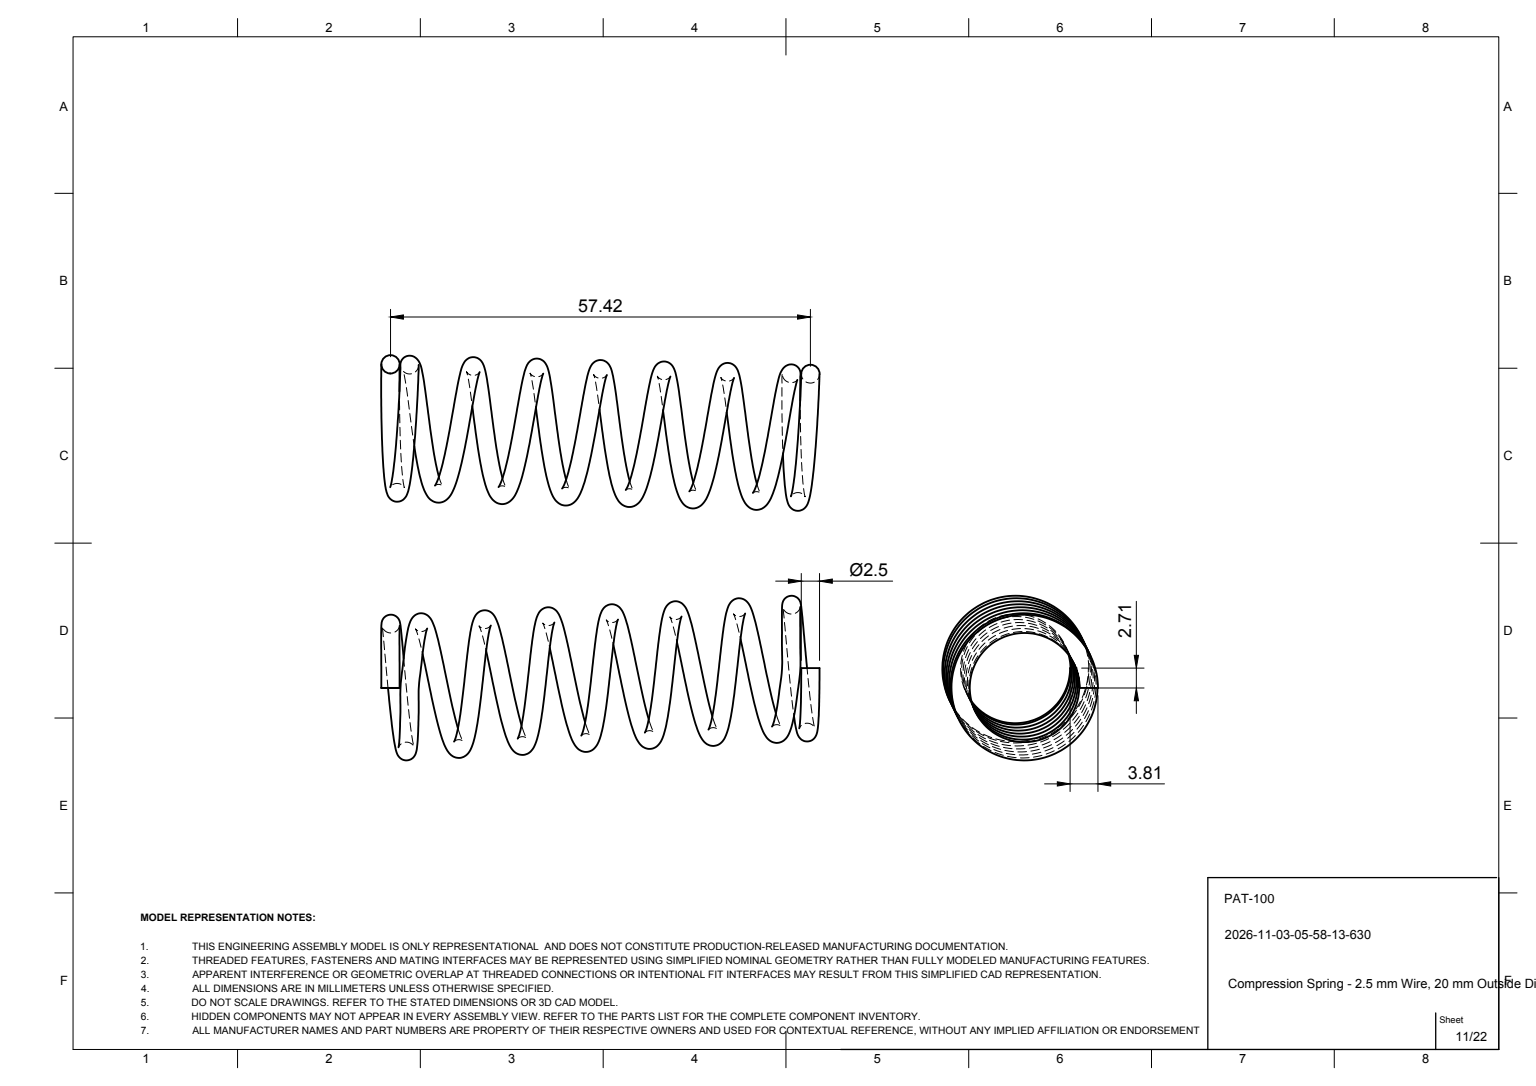
ISO-10303-21;
HEADER;
/* Generated by software containing ST-Developer
 * from STEP Tools, Inc. (www.steptools.com) 
 */

FILE_DESCRIPTION(
/* description */ (''),
/* implementation_level */ '2;1');

FILE_NAME(
/* name */ 'Compression Spring - 2.5 mm Wire, 20 mm Outside Diameter, 60 mm Long.step',
/* time_stamp */ '2026-10-29T16:43:51-07:00',
/* author */ (''),
/* organization */ (''),
/* preprocessor_version */ 'ST-DEVELOPER v20.2',
/* originating_system */ 'Autodesk Translation Framework v15.17.0.0',
/* authorisation */ '');

FILE_SCHEMA (('AUTOMOTIVE_DESIGN { 1 0 10303 214 3 1 1 }'));
ENDSEC;

DATA;
#10=MECHANICAL_DESIGN_GEOMETRIC_PRESENTATION_REPRESENTATION('',(#375),#10292);
#259=B_SPLINE_CURVE_WITH_KNOTS('',3,(#9348,#9349,#9350,#9351,#9352,#9353,
#9354,#9355,#9356,#9357,#9358,#9359,#9360,#9361,#9362,#9363,#9364,#9365,
#9366,#9367,#9368,#9369,#9370,#9371,#9372,#9373,#9374,#9375,#9376,#9377,
#9378,#9379,#9380,#9381,#9382,#9383,#9384,#9385,#9386,#9387,#9388,#9389,
#9390,#9391,#9392,#9393,#9394,#9395,#9396,#9397,#9398,#9399,#9400,#9401,
#9402,#9403,#9404,#9405,#9406,#9407,#9408,#9409,#9410,#9411,#9412,#9413,
#9414,#9415,#9416,#9417,#9418,#9419,#9420,#9421,#9422,#9423,#9424,#9425,
#9426,#9427,#9428,#9429,#9430,#9431,#9432,#9433,#9434,#9435,#9436,#9437,
#9438,#9439,#9440,#9441,#9442,#9443,#9444,#9445,#9446,#9447,#9448,#9449,
#9450,#9451,#9452,#9453,#9454,#9455,#9456,#9457,#9458,#9459,#9460,#9461,
#9462,#9463,#9464,#9465,#9466,#9467,#9468,#9469,#9470),.UNSPECIFIED.,.F.,
 .F.,(4,1,1,1,1,1,1,1,1,1,1,1,1,1,1,1,1,1,1,1,1,1,1,1,1,1,1,1,1,1,1,1,1,
1,1,1,1,1,1,1,1,1,1,1,1,1,1,1,1,1,1,1,1,1,1,1,1,1,1,1,1,1,1,1,1,1,1,1,1,
1,1,1,1,1,1,1,1,1,1,1,1,1,1,1,1,1,1,1,1,1,1,1,1,1,1,1,1,1,1,1,1,1,1,1,1,
1,1,1,1,1,1,1,1,1,1,1,1,1,1,1,4),(0.,0.00446428571428571,0.00892857142857143,
0.0178571428571429,0.0267857142857143,0.0357142857142857,0.0446428571428571,
0.0535714285714286,0.0625,0.0714285714285714,0.0803571428571428,0.0892857142857143,
0.0982142857142857,0.107142857142857,0.111607142857143,0.116071428571429,
0.120535714285714,0.122767857142857,0.125,0.129464285714286,0.133928571428571,
0.138392857142857,0.142857142857143,0.151785714285714,0.160714285714286,
0.169642857142857,0.174107142857143,0.178571428571429,0.1875,0.196428571428571,
0.205357142857143,0.214285714285714,0.223214285714286,0.232142857142857,
0.241071428571429,0.25,0.258928571428571,0.267857142857143,0.276785714285714,
0.285714285714286,0.294642857142857,0.303571428571429,0.3125,0.321428571428571,
0.330357142857143,0.339285714285714,0.348214285714286,0.357142857142857,
0.363095238095238,0.369047619047619,0.380952380952381,0.392857142857143,
0.401785714285714,0.410714285714286,0.419642857142857,0.428571428571429,
0.4375,0.446428571428571,0.455357142857143,0.464285714285714,0.476190476190476,
0.488095238095238,0.5,0.508928571428571,0.517857142857143,0.526785714285714,
0.535714285714286,0.544642857142857,0.553571428571429,0.5625,0.571428571428571,
0.580357142857143,0.589285714285714,0.598214285714286,0.607142857142857,
0.616071428571429,0.625,0.633928571428571,0.642857142857143,0.654761904761905,
0.666666666666667,0.678571428571428,0.6875,0.696428571428571,0.705357142857143,
0.714285714285714,0.720238095238095,0.726190476190476,0.738095238095238,
0.75,0.761904761904762,0.773809523809524,0.785714285714286,0.797619047619047,
0.809523809523809,0.821428571428571,0.833333333333333,0.845238095238095,
0.857142857142857,0.861607142857143,0.866071428571429,0.870535714285714,
0.875,0.877232142857143,0.879464285714286,0.883928571428571,0.888392857142857,
0.892857142857143,0.901785714285714,0.910714285714286,0.919642857142857,
0.928571428571429,0.9375,0.946428571428571,0.955357142857143,0.964285714285714,
0.973214285714286,0.982142857142857,0.991071428571429,0.995535714285714,
1.),.UNSPECIFIED.);
#264=B_SPLINE_SURFACE_WITH_KNOTS('',3,3,((#8115,#8116,#8117,#8118,#8119,
#8120,#8121,#8122,#8123,#8124,#8125,#8126,#8127,#8128,#8129,#8130,#8131,
#8132,#8133,#8134,#8135,#8136,#8137,#8138,#8139,#8140,#8141,#8142,#8143,
#8144,#8145,#8146,#8147,#8148,#8149,#8150,#8151,#8152,#8153,#8154,#8155,
#8156,#8157,#8158,#8159,#8160,#8161,#8162,#8163,#8164,#8165,#8166,#8167,
#8168,#8169,#8170,#8171,#8172,#8173,#8174,#8175,#8176,#8177,#8178,#8179,
#8180,#8181,#8182,#8183,#8184,#8185,#8186,#8187,#8188,#8189,#8190,#8191,
#8192,#8193,#8194,#8195,#8196,#8197,#8198,#8199,#8200,#8201,#8202,#8203,
#8204,#8205,#8206,#8207,#8208,#8209,#8210,#8211,#8212,#8213,#8214,#8215,
#8216,#8217,#8218,#8219,#8220,#8221,#8222,#8223,#8224,#8225,#8226,#8227,
#8228,#8229,#8230,#8231,#8232,#8233,#8234,#8235,#8236,#8237),(#8238,#8239,
#8240,#8241,#8242,#8243,#8244,#8245,#8246,#8247,#8248,#8249,#8250,#8251,
#8252,#8253,#8254,#8255,#8256,#8257,#8258,#8259,#8260,#8261,#8262,#8263,
#8264,#8265,#8266,#8267,#8268,#8269,#8270,#8271,#8272,#8273,#8274,#8275,
#8276,#8277,#8278,#8279,#8280,#8281,#8282,#8283,#8284,#8285,#8286,#8287,
#8288,#8289,#8290,#8291,#8292,#8293,#8294,#8295,#8296,#8297,#8298,#8299,
#8300,#8301,#8302,#8303,#8304,#8305,#8306,#8307,#8308,#8309,#8310,#8311,
#8312,#8313,#8314,#8315,#8316,#8317,#8318,#8319,#8320,#8321,#8322,#8323,
#8324,#8325,#8326,#8327,#8328,#8329,#8330,#8331,#8332,#8333,#8334,#8335,
#8336,#8337,#8338,#8339,#8340,#8341,#8342,#8343,#8344,#8345,#8346,#8347,
#8348,#8349,#8350,#8351,#8352,#8353,#8354,#8355,#8356,#8357,#8358,#8359,
#8360),(#8361,#8362,#8363,#8364,#8365,#8366,#8367,#8368,#8369,#8370,#8371,
#8372,#8373,#8374,#8375,#8376,#8377,#8378,#8379,#8380,#8381,#8382,#8383,
#8384,#8385,#8386,#8387,#8388,#8389,#8390,#8391,#8392,#8393,#8394,#8395,
#8396,#8397,#8398,#8399,#8400,#8401,#8402,#8403,#8404,#8405,#8406,#8407,
#8408,#8409,#8410,#8411,#8412,#8413,#8414,#8415,#8416,#8417,#8418,#8419,
#8420,#8421,#8422,#8423,#8424,#8425,#8426,#8427,#8428,#8429,#8430,#8431,
#8432,#8433,#8434,#8435,#8436,#8437,#8438,#8439,#8440,#8441,#8442,#8443,
#8444,#8445,#8446,#8447,#8448,#8449,#8450,#8451,#8452,#8453,#8454,#8455,
#8456,#8457,#8458,#8459,#8460,#8461,#8462,#8463,#8464,#8465,#8466,#8467,
#8468,#8469,#8470,#8471,#8472,#8473,#8474,#8475,#8476,#8477,#8478,#8479,
#8480,#8481,#8482,#8483),(#8484,#8485,#8486,#8487,#8488,#8489,#8490,#8491,
#8492,#8493,#8494,#8495,#8496,#8497,#8498,#8499,#8500,#8501,#8502,#8503,
#8504,#8505,#8506,#8507,#8508,#8509,#8510,#8511,#8512,#8513,#8514,#8515,
#8516,#8517,#8518,#8519,#8520,#8521,#8522,#8523,#8524,#8525,#8526,#8527,
#8528,#8529,#8530,#8531,#8532,#8533,#8534,#8535,#8536,#8537,#8538,#8539,
#8540,#8541,#8542,#8543,#8544,#8545,#8546,#8547,#8548,#8549,#8550,#8551,
#8552,#8553,#8554,#8555,#8556,#8557,#8558,#8559,#8560,#8561,#8562,#8563,
#8564,#8565,#8566,#8567,#8568,#8569,#8570,#8571,#8572,#8573,#8574,#8575,
#8576,#8577,#8578,#8579,#8580,#8581,#8582,#8583,#8584,#8585,#8586,#8587,
#8588,#8589,#8590,#8591,#8592,#8593,#8594,#8595,#8596,#8597,#8598,#8599,
#8600,#8601,#8602,#8603,#8604,#8605,#8606),(#8607,#8608,#8609,#8610,#8611,
#8612,#8613,#8614,#8615,#8616,#8617,#8618,#8619,#8620,#8621,#8622,#8623,
#8624,#8625,#8626,#8627,#8628,#8629,#8630,#8631,#8632,#8633,#8634,#8635,
#8636,#8637,#8638,#8639,#8640,#8641,#8642,#8643,#8644,#8645,#8646,#8647,
#8648,#8649,#8650,#8651,#8652,#8653,#8654,#8655,#8656,#8657,#8658,#8659,
#8660,#8661,#8662,#8663,#8664,#8665,#8666,#8667,#8668,#8669,#8670,#8671,
#8672,#8673,#8674,#8675,#8676,#8677,#8678,#8679,#8680,#8681,#8682,#8683,
#8684,#8685,#8686,#8687,#8688,#8689,#8690,#8691,#8692,#8693,#8694,#8695,
#8696,#8697,#8698,#8699,#8700,#8701,#8702,#8703,#8704,#8705,#8706,#8707,
#8708,#8709,#8710,#8711,#8712,#8713,#8714,#8715,#8716,#8717,#8718,#8719,
#8720,#8721,#8722,#8723,#8724,#8725,#8726,#8727,#8728,#8729),(#8730,#8731,
#8732,#8733,#8734,#8735,#8736,#8737,#8738,#8739,#8740,#8741,#8742,#8743,
#8744,#8745,#8746,#8747,#8748,#8749,#8750,#8751,#8752,#8753,#8754,#8755,
#8756,#8757,#8758,#8759,#8760,#8761,#8762,#8763,#8764,#8765,#8766,#8767,
#8768,#8769,#8770,#8771,#8772,#8773,#8774,#8775,#8776,#8777,#8778,#8779,
#8780,#8781,#8782,#8783,#8784,#8785,#8786,#8787,#8788,#8789,#8790,#8791,
#8792,#8793,#8794,#8795,#8796,#8797,#8798,#8799,#8800,#8801,#8802,#8803,
#8804,#8805,#8806,#8807,#8808,#8809,#8810,#8811,#8812,#8813,#8814,#8815,
#8816,#8817,#8818,#8819,#8820,#8821,#8822,#8823,#8824,#8825,#8826,#8827,
#8828,#8829,#8830,#8831,#8832,#8833,#8834,#8835,#8836,#8837,#8838,#8839,
#8840,#8841,#8842,#8843,#8844,#8845,#8846,#8847,#8848,#8849,#8850,#8851,
#8852),(#8853,#8854,#8855,#8856,#8857,#8858,#8859,#8860,#8861,#8862,#8863,
#8864,#8865,#8866,#8867,#8868,#8869,#8870,#8871,#8872,#8873,#8874,#8875,
#8876,#8877,#8878,#8879,#8880,#8881,#8882,#8883,#8884,#8885,#8886,#8887,
#8888,#8889,#8890,#8891,#8892,#8893,#8894,#8895,#8896,#8897,#8898,#8899,
#8900,#8901,#8902,#8903,#8904,#8905,#8906,#8907,#8908,#8909,#8910,#8911,
#8912,#8913,#8914,#8915,#8916,#8917,#8918,#8919,#8920,#8921,#8922,#8923,
#8924,#8925,#8926,#8927,#8928,#8929,#8930,#8931,#8932,#8933,#8934,#8935,
#8936,#8937,#8938,#8939,#8940,#8941,#8942,#8943,#8944,#8945,#8946,#8947,
#8948,#8949,#8950,#8951,#8952,#8953,#8954,#8955,#8956,#8957,#8958,#8959,
#8960,#8961,#8962,#8963,#8964,#8965,#8966,#8967,#8968,#8969,#8970,#8971,
#8972,#8973,#8974,#8975),(#8976,#8977,#8978,#8979,#8980,#8981,#8982,#8983,
#8984,#8985,#8986,#8987,#8988,#8989,#8990,#8991,#8992,#8993,#8994,#8995,
#8996,#8997,#8998,#8999,#9000,#9001,#9002,#9003,#9004,#9005,#9006,#9007,
#9008,#9009,#9010,#9011,#9012,#9013,#9014,#9015,#9016,#9017,#9018,#9019,
#9020,#9021,#9022,#9023,#9024,#9025,#9026,#9027,#9028,#9029,#9030,#9031,
#9032,#9033,#9034,#9035,#9036,#9037,#9038,#9039,#9040,#9041,#9042,#9043,
#9044,#9045,#9046,#9047,#9048,#9049,#9050,#9051,#9052,#9053,#9054,#9055,
#9056,#9057,#9058,#9059,#9060,#9061,#9062,#9063,#9064,#9065,#9066,#9067,
#9068,#9069,#9070,#9071,#9072,#9073,#9074,#9075,#9076,#9077,#9078,#9079,
#9080,#9081,#9082,#9083,#9084,#9085,#9086,#9087,#9088,#9089,#9090,#9091,
#9092,#9093,#9094,#9095,#9096,#9097,#9098),(#9099,#9100,#9101,#9102,#9103,
#9104,#9105,#9106,#9107,#9108,#9109,#9110,#9111,#9112,#9113,#9114,#9115,
#9116,#9117,#9118,#9119,#9120,#9121,#9122,#9123,#9124,#9125,#9126,#9127,
#9128,#9129,#9130,#9131,#9132,#9133,#9134,#9135,#9136,#9137,#9138,#9139,
#9140,#9141,#9142,#9143,#9144,#9145,#9146,#9147,#9148,#9149,#9150,#9151,
#9152,#9153,#9154,#9155,#9156,#9157,#9158,#9159,#9160,#9161,#9162,#9163,
#9164,#9165,#9166,#9167,#9168,#9169,#9170,#9171,#9172,#9173,#9174,#9175,
#9176,#9177,#9178,#9179,#9180,#9181,#9182,#9183,#9184,#9185,#9186,#9187,
#9188,#9189,#9190,#9191,#9192,#9193,#9194,#9195,#9196,#9197,#9198,#9199,
#9200,#9201,#9202,#9203,#9204,#9205,#9206,#9207,#9208,#9209,#9210,#9211,
#9212,#9213,#9214,#9215,#9216,#9217,#9218,#9219,#9220,#9221),(#9222,#9223,
#9224,#9225,#9226,#9227,#9228,#9229,#9230,#9231,#9232,#9233,#9234,#9235,
#9236,#9237,#9238,#9239,#9240,#9241,#9242,#9243,#9244,#9245,#9246,#9247,
#9248,#9249,#9250,#9251,#9252,#9253,#9254,#9255,#9256,#9257,#9258,#9259,
#9260,#9261,#9262,#9263,#9264,#9265,#9266,#9267,#9268,#9269,#9270,#9271,
#9272,#9273,#9274,#9275,#9276,#9277,#9278,#9279,#9280,#9281,#9282,#9283,
#9284,#9285,#9286,#9287,#9288,#9289,#9290,#9291,#9292,#9293,#9294,#9295,
#9296,#9297,#9298,#9299,#9300,#9301,#9302,#9303,#9304,#9305,#9306,#9307,
#9308,#9309,#9310,#9311,#9312,#9313,#9314,#9315,#9316,#9317,#9318,#9319,
#9320,#9321,#9322,#9323,#9324,#9325,#9326,#9327,#9328,#9329,#9330,#9331,
#9332,#9333,#9334,#9335,#9336,#9337,#9338,#9339,#9340,#9341,#9342,#9343,
#9344)),.UNSPECIFIED.,.T.,.F.,.F.,(4,1,1,1,1,1,1,4),(4,1,1,1,1,1,1,1,1,
1,1,1,1,1,1,1,1,1,1,1,1,1,1,1,1,1,1,1,1,1,1,1,1,1,1,1,1,1,1,1,1,1,1,1,1,
1,1,1,1,1,1,1,1,1,1,1,1,1,1,1,1,1,1,1,1,1,1,1,1,1,1,1,1,1,1,1,1,1,1,1,1,
1,1,1,1,1,1,1,1,1,1,1,1,1,1,1,1,1,1,1,1,1,1,1,1,1,1,1,1,1,1,1,1,1,1,1,1,
1,1,1,4),(-3.14159265358979,-2.24399475256414,-1.34639685153848,-0.448798950512828,
0.448798950512828,1.34639685153848,2.24399475256414,3.14159265358979),(0.,
0.00446428571428571,0.00892857142857143,0.0178571428571429,0.0267857142857143,
0.0357142857142857,0.0446428571428571,0.0535714285714286,0.0625,0.0714285714285714,
0.0803571428571428,0.0892857142857143,0.0982142857142857,0.107142857142857,
0.111607142857143,0.116071428571429,0.120535714285714,0.122767857142857,
0.125,0.129464285714286,0.133928571428571,0.138392857142857,0.142857142857143,
0.151785714285714,0.160714285714286,0.169642857142857,0.174107142857143,
0.178571428571429,0.1875,0.196428571428571,0.205357142857143,0.214285714285714,
0.223214285714286,0.232142857142857,0.241071428571429,0.25,0.258928571428571,
0.267857142857143,0.276785714285714,0.285714285714286,0.294642857142857,
0.303571428571429,0.3125,0.321428571428571,0.330357142857143,0.339285714285714,
0.348214285714286,0.357142857142857,0.363095238095238,0.369047619047619,
0.380952380952381,0.392857142857143,0.401785714285714,0.410714285714286,
0.419642857142857,0.428571428571429,0.4375,0.446428571428571,0.455357142857143,
0.464285714285714,0.476190476190476,0.488095238095238,0.5,0.508928571428571,
0.517857142857143,0.526785714285714,0.535714285714286,0.544642857142857,
0.553571428571429,0.5625,0.571428571428571,0.580357142857143,0.589285714285714,
0.598214285714286,0.607142857142857,0.616071428571429,0.625,0.633928571428571,
0.642857142857143,0.654761904761905,0.666666666666667,0.678571428571428,
0.6875,0.696428571428571,0.705357142857143,0.714285714285714,0.720238095238095,
0.726190476190476,0.738095238095238,0.75,0.761904761904762,0.773809523809524,
0.785714285714286,0.797619047619047,0.809523809523809,0.821428571428571,
0.833333333333333,0.845238095238095,0.857142857142857,0.861607142857143,
0.866071428571429,0.870535714285714,0.875,0.877232142857143,0.879464285714286,
0.883928571428571,0.888392857142857,0.892857142857143,0.901785714285714,
0.910714285714286,0.919642857142857,0.928571428571429,0.9375,0.946428571428571,
0.955357142857143,0.964285714285714,0.973214285714286,0.982142857142857,
0.991071428571429,0.995535714285714,1.),.UNSPECIFIED.);
#329=SHAPE_REPRESENTATION_RELATIONSHIP('SRR','None',#10425,#352);
#352=ADVANCED_BREP_SHAPE_REPRESENTATION('',(#396),#10277);
#375=STYLED_ITEM('',(#10628),#396);
#396=MANIFOLD_SOLID_BREP('Body1',#5019);
#619=PLANE('',#5533);
#620=PLANE('',#5534);
#849=FACE_OUTER_BOUND('',#1201,.T.);
#850=FACE_OUTER_BOUND('',#1202,.T.);
#851=FACE_OUTER_BOUND('',#1203,.T.);
#1201=EDGE_LOOP('',(#4039,#4040,#4041,#4042));
#1202=EDGE_LOOP('',(#4043));
#1203=EDGE_LOOP('',(#4044));
#2285=CIRCLE('',#5531,0.125);
#2286=CIRCLE('',#5532,0.125);
#2600=VERTEX_POINT('',#9345);
#2601=VERTEX_POINT('',#9347);
#3110=EDGE_CURVE('',#2600,#2600,#2285,.T.);
#3111=EDGE_CURVE('',#2600,#2601,#259,.T.);
#3112=EDGE_CURVE('',#2601,#2601,#2286,.T.);
#4039=ORIENTED_EDGE('',*,*,#3110,.T.);
#4040=ORIENTED_EDGE('',*,*,#3111,.T.);
#4041=ORIENTED_EDGE('',*,*,#3112,.F.);
#4042=ORIENTED_EDGE('',*,*,#3111,.F.);
#4043=ORIENTED_EDGE('',*,*,#3112,.T.);
#4044=ORIENTED_EDGE('',*,*,#3110,.F.);
#4858=ADVANCED_FACE('',(#849),#264,.T.);
#4859=ADVANCED_FACE('',(#850),#619,.T.);
#4860=ADVANCED_FACE('',(#851),#620,.F.);
#5019=CLOSED_SHELL('',(#4858,#4859,#4860));
#5530=AXIS2_PLACEMENT_3D('',#8114,#6553,#6554);
#5531=AXIS2_PLACEMENT_3D('',#9346,#6555,#6556);
#5532=AXIS2_PLACEMENT_3D('',#9471,#6557,#6558);
#5533=AXIS2_PLACEMENT_3D('',#9472,#6559,#6560);
#5534=AXIS2_PLACEMENT_3D('',#9473,#6561,#6562);
#6553=DIRECTION('axis',(0.,0.,1.));
#6554=DIRECTION('refdir',(1.,0.,0.));
#6555=DIRECTION('center_axis',(-0.00107151163471255,0.0471293712697611,
0.998888219084865));
#6556=DIRECTION('ref_axis',(0.022704394310356,-0.998630154113891,0.0471415503931119));
#6557=DIRECTION('center_axis',(0.0010715115821705,0.0471293712204561,0.998888219087248));
#6558=DIRECTION('ref_axis',(0.234516922063796,-0.971043629832377,0.045564045339339));
#6559=DIRECTION('center_axis',(0.0010715115821705,0.0471293712204561,0.998888219087248));
#6560=DIRECTION('ref_axis',(0.234516922063796,-0.971043629832377,0.045564045339339));
#6561=DIRECTION('center_axis',(-0.00107151163471255,0.0471293712697611,
0.998888219084865));
#6562=DIRECTION('ref_axis',(0.022704394310356,-0.998630154113891,0.0471415503931119));
#8114=CARTESIAN_POINT('',(0.,0.,0.));
#8115=CARTESIAN_POINT('Ctrl Pts',(0.872161950711206,0.124828769264236,-0.00589269379913899));
#8116=CARTESIAN_POINT('Ctrl Pts',(0.872090904698941,0.127953657301625,0.0603380612992187));
#8117=CARTESIAN_POINT('Ctrl Pts',(0.857308714561314,0.134203213047992,0.190241275757611));
#8118=CARTESIAN_POINT('Ctrl Pts',(0.770187083636269,0.146690001256174,0.438769378299054));
#8119=CARTESIAN_POINT('Ctrl Pts',(0.560950745207346,0.162256028321672,0.699616259986153));
#8120=CARTESIAN_POINT('Ctrl Pts',(0.199511576340965,0.180880209711553,0.871422024437173));
#8121=CARTESIAN_POINT('Ctrl Pts',(-0.199312333389545,0.199448331926636,
0.868457819907934));
#8122=CARTESIAN_POINT('Ctrl Pts',(-0.556088930421348,0.217951986567579,
0.692928582783942));
#8123=CARTESIAN_POINT('Ctrl Pts',(-0.799862508003898,0.236416030436661,
0.380262416576452));
#8124=CARTESIAN_POINT('Ctrl Pts',(-0.882895646021795,0.254773193569333,
-0.0060546706614528));
#8125=CARTESIAN_POINT('Ctrl Pts',(-0.789649057445972,0.273182184223599,
-0.388883291654368));
#8126=CARTESIAN_POINT('Ctrl Pts',(-0.539659944242912,0.291280837799174,
-0.691764713311758));
#8127=CARTESIAN_POINT('Ctrl Pts',(-0.183956800223335,0.309860445327341,
-0.855316888413074));
#8128=CARTESIAN_POINT('Ctrl Pts',(0.206499015809491,0.327389549600143,-0.847162298078497));
#8129=CARTESIAN_POINT('Ctrl Pts',(0.49509577120488,0.34362645645855,-0.700495805282282));
#8130=CARTESIAN_POINT('Ctrl Pts',(0.670997034604971,0.353943958171212,-0.515417881277946));
#8131=CARTESIAN_POINT('Ctrl Pts',(0.766581438347442,0.365141873832304,-0.355537227212008));
#8132=CARTESIAN_POINT('Ctrl Pts',(0.8174676017473,0.371459915026287,-0.198233634126398));
#8133=CARTESIAN_POINT('Ctrl Pts',(0.834170515466371,0.374539492519685,-0.0771620442826736));
#8134=CARTESIAN_POINT('Ctrl Pts',(0.837719002104484,0.383704512647053,0.0354460071939376));
#8135=CARTESIAN_POINT('Ctrl Pts',(0.817405541799073,0.413175723298386,0.185924750839524));
#8136=CARTESIAN_POINT('Ctrl Pts',(0.748423543506377,0.44312071842525,0.367957985006333));
#8137=CARTESIAN_POINT('Ctrl Pts',(0.647340094288683,0.470691270109384,0.518903872562794));
#8138=CARTESIAN_POINT('Ctrl Pts',(0.466898254116811,0.511144063135416,0.691309623343175));
#8139=CARTESIAN_POINT('Ctrl Pts',(0.182800989155019,0.558222951408999,0.818397523700333));
#8140=CARTESIAN_POINT('Ctrl Pts',(-0.189545178060892,0.616501258086875,
0.809773850041606));
#8141=CARTESIAN_POINT('Ctrl Pts',(-0.462507583347405,0.663503908067788,
0.669357773844709));
#8142=CARTESIAN_POINT('Ctrl Pts',(-0.627863189228003,0.701318402481341,
0.495969553901588));
#8143=CARTESIAN_POINT('Ctrl Pts',(-0.750267427503473,0.738837453517587,
0.291088758101646));
#8144=CARTESIAN_POINT('Ctrl Pts',(-0.810712868559922,0.785528896923523,
-0.00492588128797676));
#8145=CARTESIAN_POINT('Ctrl Pts',(-0.722807305049749,0.841109138477463,
-0.35397737605765));
#8146=CARTESIAN_POINT('Ctrl Pts',(-0.493845277109899,0.896322143289524,
-0.6284699970223));
#8147=CARTESIAN_POINT('Ctrl Pts',(-0.170668331595556,0.951180240767939,
-0.77578162036287));
#8148=CARTESIAN_POINT('Ctrl Pts',(0.182411368712431,1.00572789901627,-0.768554583075931));
#8149=CARTESIAN_POINT('Ctrl Pts',(0.495894675031221,1.0599979812032,-0.609891173973463));
#8150=CARTESIAN_POINT('Ctrl Pts',(0.708755333326572,1.11403086100534,-0.332295680974433));
#8151=CARTESIAN_POINT('Ctrl Pts',(0.780070637830783,1.16786510347237,0.00885468431853584));
#8152=CARTESIAN_POINT('Ctrl Pts',(0.696791510479646,1.22154183082612,0.346232027663686));
#8153=CARTESIAN_POINT('Ctrl Pts',(0.476047266626745,1.27510240963086,0.61364355273423));
#8154=CARTESIAN_POINT('Ctrl Pts',(0.161678386661078,1.32858888114584,0.758820094473604));
#8155=CARTESIAN_POINT('Ctrl Pts',(-0.184345221885054,1.38204344182885,0.753472314023915));
#8156=CARTESIAN_POINT('Ctrl Pts',(-0.493955884546455,1.43550888318168,0.598711183433611));
#8157=CARTESIAN_POINT('Ctrl Pts',(-0.706164418456796,1.48902767046263,0.324820470310737));
#8158=CARTESIAN_POINT('Ctrl Pts',(-0.778894190579621,1.54264192169839,-0.0145743797186695));
#8159=CARTESIAN_POINT('Ctrl Pts',(-0.697192877485004,1.59639341722752,-0.352835018065878));
#8160=CARTESIAN_POINT('Ctrl Pts',(-0.476282548914222,1.65032345266182,-0.623209180930827));
#8161=CARTESIAN_POINT('Ctrl Pts',(-0.158743612035258,1.70447207761938,-0.771770092812482));
#8162=CARTESIAN_POINT('Ctrl Pts',(0.193450677004803,1.75887837965647,-0.768113401787862));
#8163=CARTESIAN_POINT('Ctrl Pts',(0.47579440943534,1.80750241451549,-0.628734440560694));
#8164=CARTESIAN_POINT('Ctrl Pts',(0.659272267850805,1.85026369378763,-0.426676852570877));
#8165=CARTESIAN_POINT('Ctrl Pts',(0.793229432459306,1.89934423589563,-0.143355198493509));
#8166=CARTESIAN_POINT('Ctrl Pts',(0.790263784307131,1.96111512092083,0.264407243055348));
#8167=CARTESIAN_POINT('Ctrl Pts',(0.532639208585251,2.02974904747753,0.637020032041957));
#8168=CARTESIAN_POINT('Ctrl Pts',(0.163609475192015,2.09273970975414,0.811198964310618));
#8169=CARTESIAN_POINT('Ctrl Pts',(-0.206325324489528,2.14991769756873,0.809290051602918));
#8170=CARTESIAN_POINT('Ctrl Pts',(-0.54210311156644,2.20760646525503,0.645493293137588));
#8171=CARTESIAN_POINT('Ctrl Pts',(-0.775793177879044,2.26582771180786,0.349801965195082));
#8172=CARTESIAN_POINT('Ctrl Pts',(-0.859118193146955,2.32460053758821,-0.0214433086745682));
#8173=CARTESIAN_POINT('Ctrl Pts',(-0.772497333242961,2.38394137391289,-0.395836964477112));
#8174=CARTESIAN_POINT('Ctrl Pts',(-0.529877815574135,2.44386394296014,-0.698375208084907));
#8175=CARTESIAN_POINT('Ctrl Pts',(-0.137454124419672,2.51110274201743,-0.887126219786336));
#8176=CARTESIAN_POINT('Ctrl Pts',(0.355020405406913,2.58592160387692,-0.85044216028401));
#8177=CARTESIAN_POINT('Ctrl Pts',(0.782180417385646,2.66862024366749,-0.50996194705241));
#8178=CARTESIAN_POINT('Ctrl Pts',(0.932029131507338,2.74541647960869,-0.0258957186176781));
#8179=CARTESIAN_POINT('Ctrl Pts',(0.830321215974015,2.81601192011723,0.419957402046343));
#8180=CARTESIAN_POINT('Ctrl Pts',(0.572400166827825,2.88014282443316,0.744989944459363));
#8181=CARTESIAN_POINT('Ctrl Pts',(0.195275509838113,2.94485897026784,0.927771382562365));
#8182=CARTESIAN_POINT('Ctrl Pts',(-0.227340767365424,3.01014754818103,0.929095017890615));
#8183=CARTESIAN_POINT('Ctrl Pts',(-0.612127646814787,3.07599293903656,0.745588291188903));
#8184=CARTESIAN_POINT('Ctrl Pts',(-0.881535208369304,3.14237676662695,0.410744646425331));
#8185=CARTESIAN_POINT('Ctrl Pts',(-0.980005185206354,3.20927820175596,-0.0110388926131081));
#8186=CARTESIAN_POINT('Ctrl Pts',(-0.885263395772081,3.27667359822412,-0.436952466191731));
#8187=CARTESIAN_POINT('Ctrl Pts',(-0.613436538369041,3.34453700325931,-0.782121048029494));
#8188=CARTESIAN_POINT('Ctrl Pts',(-0.216315847404239,3.41284022102408,-0.976638893510757));
#8189=CARTESIAN_POINT('Ctrl Pts',(0.228515688692952,3.48155290325642,-0.979879367890244));
#8190=CARTESIAN_POINT('Ctrl Pts',(0.633032334246116,3.55064249055004,-0.788946617304531));
#8191=CARTESIAN_POINT('Ctrl Pts',(0.91620307923501,3.62007471455624,-0.439929095068272));
#8192=CARTESIAN_POINT('Ctrl Pts',(1.02068551154318,3.6898138200776,-0.00055988972616793));
#8193=CARTESIAN_POINT('Ctrl Pts',(0.923874643413053,3.75982214337787,0.441983752855437));
#8194=CARTESIAN_POINT('Ctrl Pts',(0.613247660943624,3.83786518922612,0.840785019888275));
#8195=CARTESIAN_POINT('Ctrl Pts',(0.0866578234258063,3.9239844102579,1.05456997463629));
#8196=CARTESIAN_POINT('Ctrl Pts',(-0.521392660403112,4.01817435387289,0.92294994186792));
#8197=CARTESIAN_POINT('Ctrl Pts',(-0.914636612404499,4.10464567111125,0.509573712510557));
#8198=CARTESIAN_POINT('Ctrl Pts',(-1.03374180999006,4.18328650371776,0.0141535738014065));
#8199=CARTESIAN_POINT('Ctrl Pts',(-0.938026942329867,4.25404428614242,-0.433573776623787));
#8200=CARTESIAN_POINT('Ctrl Pts',(-0.657630260146868,4.32474041714926,-0.795496981882739));
#8201=CARTESIAN_POINT('Ctrl Pts',(-0.294187702113077,4.38748944604847,-0.977023505420508));
#8202=CARTESIAN_POINT('Ctrl Pts',(0.0542596632323615,4.44230054898675,-1.00807090756588));
#8203=CARTESIAN_POINT('Ctrl Pts',(0.445198581282316,4.50483969839108,-0.926094625208896));
#8204=CARTESIAN_POINT('Ctrl Pts',(0.852563310440807,4.58279123657346,-0.611941112564204));
#8205=CARTESIAN_POINT('Ctrl Pts',(1.04336115553597,4.67588518836249,-0.0274765552718303));
#8206=CARTESIAN_POINT('Ctrl Pts',(0.873243552350396,4.76843871793217,0.559396655291762));
#8207=CARTESIAN_POINT('Ctrl Pts',(0.405532574611691,4.86037265153526,0.946224142384314));
#8208=CARTESIAN_POINT('Ctrl Pts',(-0.194232561825003,4.95159408982323,1.00246182575268));
#8209=CARTESIAN_POINT('Ctrl Pts',(-0.716978005254575,5.04205915598986,0.713684974901636));
#8210=CARTESIAN_POINT('Ctrl Pts',(-0.984237521133288,5.13163619116299,0.185945073380498));
#8211=CARTESIAN_POINT('Ctrl Pts',(-0.909022704364039,5.22040809154829,-0.394980663551699));
#8212=CARTESIAN_POINT('Ctrl Pts',(-0.524008362921299,5.30799616173538,-0.827628543573509));
#8213=CARTESIAN_POINT('Ctrl Pts',(0.0311612934979211,5.39510126764713,-0.968284503878036));
#8214=CARTESIAN_POINT('Ctrl Pts',(0.452486451456519,5.46227744588555,-0.812413771015693));
#8215=CARTESIAN_POINT('Ctrl Pts',(0.678996914481602,5.51263767773254,-0.597335976683866));
#8216=CARTESIAN_POINT('Ctrl Pts',(0.792756702852497,5.54424482065645,-0.425194580715441));
#8217=CARTESIAN_POINT('Ctrl Pts',(0.861097079444627,5.57344984716716,-0.244943323368279));
#8218=CARTESIAN_POINT('Ctrl Pts',(0.885548394683697,5.6069898998326,-0.0758116878038518));
#8219=CARTESIAN_POINT('Ctrl Pts',(0.881311178103886,5.61908885250671,0.0702661570768112));
#8220=CARTESIAN_POINT('Ctrl Pts',(0.861324400417122,5.62225654974902,0.205633030471336));
#8221=CARTESIAN_POINT('Ctrl Pts',(0.812891366893097,5.62852110126019,0.357273663598819));
#8222=CARTESIAN_POINT('Ctrl Pts',(0.709033945858278,5.64053429758327,0.532105911493553));
#8223=CARTESIAN_POINT('Ctrl Pts',(0.526480038594941,5.65124067536637,0.723242801555853));
#8224=CARTESIAN_POINT('Ctrl Pts',(0.225331281496905,5.66829963228703,0.876812377650357));
#8225=CARTESIAN_POINT('Ctrl Pts',(-0.178438754359568,5.6861889761217,0.884400172818289));
#8226=CARTESIAN_POINT('Ctrl Pts',(-0.544244744848784,5.70539124964099,0.716342713969011));
#8227=CARTESIAN_POINT('Ctrl Pts',(-0.799436178683323,5.72389218103035,0.406445379440496));
#8228=CARTESIAN_POINT('Ctrl Pts',(-0.893901515434013,5.74261482334007,0.0176118727011753));
#8229=CARTESIAN_POINT('Ctrl Pts',(-0.809793026073925,5.76114914213192,-0.372336066624544));
#8230=CARTESIAN_POINT('Ctrl Pts',(-0.565009292976944,5.77968086993593,-0.685823620580416));
#8231=CARTESIAN_POINT('Ctrl Pts',(-0.209171565907703,5.79813086800354,-0.860593511818846));
#8232=CARTESIAN_POINT('Ctrl Pts',(0.186034384156284,5.8165319894943,-0.863241242665013));
#8233=CARTESIAN_POINT('Ctrl Pts',(0.541844299347737,5.83487223159308,-0.693819904186464));
#8234=CARTESIAN_POINT('Ctrl Pts',(0.746471713940332,5.85010991085684,-0.43833815015316));
#8235=CARTESIAN_POINT('Ctrl Pts',(0.831270497111571,5.86227119228351,-0.19628398706425));
#8236=CARTESIAN_POINT('Ctrl Pts',(0.845616258369985,5.86833999900766,-0.0701367303899257));
#8237=CARTESIAN_POINT('Ctrl Pts',(0.845685384742026,5.87138045372904,-0.00569550566726366));
#8238=CARTESIAN_POINT('Ctrl Pts',(0.834771700518231,0.123978681791665,-0.00589269379913899));
#8239=CARTESIAN_POINT('Ctrl Pts',(0.834703585425039,0.126974656274918,0.0576057899568015));
#8240=CARTESIAN_POINT('Ctrl Pts',(0.820566864806215,0.132951747306104,0.1818462773769));
#8241=CARTESIAN_POINT('Ctrl Pts',(0.737159418128638,0.144907869145536,0.41981635707622));
#8242=CARTESIAN_POINT('Ctrl Pts',(0.536913029824937,0.159802973361417,0.669408868982891));
#8243=CARTESIAN_POINT('Ctrl Pts',(0.19099562145444,0.177628187211079,0.833856980367138));
#8244=CARTESIAN_POINT('Ctrl Pts',(-0.190655324048718,0.195396044249228,
0.830996898689714));
#8245=CARTESIAN_POINT('Ctrl Pts',(-0.53207161478927,0.213103379696006,0.663031596529677));
#8246=CARTESIAN_POINT('Ctrl Pts',(-0.765333292231674,0.230771512020908,
0.36382917330982));
#8247=CARTESIAN_POINT('Ctrl Pts',(-0.844788059380974,0.248338044161933,
-0.00584534341205808));
#8248=CARTESIAN_POINT('Ctrl Pts',(-0.755550469517709,0.265954744653817,
-0.372189649298638));
#8249=CARTESIAN_POINT('Ctrl Pts',(-0.516314131999674,0.283275239097253,
-0.662046752944101));
#8250=CARTESIAN_POINT('Ctrl Pts',(-0.175874814910529,0.301058416266183,
-0.818563370277865));
#8251=CARTESIAN_POINT('Ctrl Pts',(0.197837874836819,0.317836237075745,-0.810772944672516));
#8252=CARTESIAN_POINT('Ctrl Pts',(0.474117448088369,0.333381343729803,-0.670340422853212));
#8253=CARTESIAN_POINT('Ctrl Pts',(0.642476318144299,0.343257359612203,-0.493219944846032));
#8254=CARTESIAN_POINT('Ctrl Pts',(0.734084644784475,0.353986453186565,-0.339953181467585));
#8255=CARTESIAN_POINT('Ctrl Pts',(0.782670889327258,0.360026050725482,-0.189705341255422));
#8256=CARTESIAN_POINT('Ctrl Pts',(0.798724557788542,0.362974904968381,-0.0735631332743304));
#8257=CARTESIAN_POINT('Ctrl Pts',(0.802141543715252,0.371811933026709,0.0349840749294869));
#8258=CARTESIAN_POINT('Ctrl Pts',(0.782571839931757,0.400140924438028,0.179601073342154));
#8259=CARTESIAN_POINT('Ctrl Pts',(0.716586436607174,0.428773049861363,0.353720744375737));
#8260=CARTESIAN_POINT('Ctrl Pts',(0.619452048298751,0.455282772577966,0.498840903387784));
#8261=CARTESIAN_POINT('Ctrl Pts',(0.446338986242718,0.494085589245527,0.664198743741128));
#8262=CARTESIAN_POINT('Ctrl Pts',(0.173348026654919,0.539339087364759,0.786420950987734));
#8263=CARTESIAN_POINT('Ctrl Pts',(-0.184821452882668,0.595395544254175,
0.778115761403682));
#8264=CARTESIAN_POINT('Ctrl Pts',(-0.447871399056696,0.640697053109364,
0.642894143294883));
#8265=CARTESIAN_POINT('Ctrl Pts',(-0.607392342756213,0.677176186867957,
0.47562801903027));
#8266=CARTESIAN_POINT('Ctrl Pts',(-0.725592115215377,0.713406676016781,
0.277808215850071));
#8267=CARTESIAN_POINT('Ctrl Pts',(-0.784113311361799,0.758571100411465,
-0.0084746015749381));
#8268=CARTESIAN_POINT('Ctrl Pts',(-0.698996863957015,0.812438504258161,
-0.346766060602901));
#8269=CARTESIAN_POINT('Ctrl Pts',(-0.476612351424375,0.866092299597088,
-0.613526369115138));
#8270=CARTESIAN_POINT('Ctrl Pts',(-0.161859501263566,0.919532790752191,
-0.757098553956881));
#8271=CARTESIAN_POINT('Ctrl Pts',(0.183015403440875,0.972820718761726,-0.750147817033866));
#8272=CARTESIAN_POINT('Ctrl Pts',(0.490154877552902,1.02599129588717,-0.59481688084477));
#8273=CARTESIAN_POINT('Ctrl Pts',(0.699403601519287,1.07909221978425,-0.322121854432755));
#8274=CARTESIAN_POINT('Ctrl Pts',(0.769817441643044,1.13216585492274,0.0141331161359554));
#8275=CARTESIAN_POINT('Ctrl Pts',(0.687578814649516,1.18525747666464,0.347809311925023));
#8276=CARTESIAN_POINT('Ctrl Pts',(0.468644093923167,1.23841119165469,0.613227239522894));
#8277=CARTESIAN_POINT('Ctrl Pts',(0.155712125133277,1.29167111889997,0.757881850017962));
#8278=CARTESIAN_POINT('Ctrl Pts',(-0.189963695061651,1.34508056439839,0.752669618582056));
#8279=CARTESIAN_POINT('Ctrl Pts',(-0.500371056919822,1.39868255819304,0.597656322850705));
#8280=CARTESIAN_POINT('Ctrl Pts',(-0.713905011413384,1.45251897515664,0.322267362968876));
#8281=CARTESIAN_POINT('Ctrl Pts',(-0.787422097915162,1.50663031435001,-0.0201881452818813));
#8282=CARTESIAN_POINT('Ctrl Pts',(-0.70483144226016,1.56105630602259,-0.362661071536256));
#8283=CARTESIAN_POINT('Ctrl Pts',(-0.480579928801225,1.61583446556222,-0.637316626417315));
#8284=CARTESIAN_POINT('Ctrl Pts',(-0.157171190478558,1.67100240976954,-0.788747246876486));
#8285=CARTESIAN_POINT('Ctrl Pts',(0.202622739833848,1.7265916485172,-0.785124172182557));
#8286=CARTESIAN_POINT('Ctrl Pts',(0.491912328391669,1.77641473527713,-0.642420818797231));
#8287=CARTESIAN_POINT('Ctrl Pts',(0.680285980292682,1.82031497486235,-0.435026313679016));
#8288=CARTESIAN_POINT('Ctrl Pts',(0.818038947603602,1.87077846101778,-0.143766162147066));
#8289=CARTESIAN_POINT('Ctrl Pts',(0.815175070026228,1.93444545082108,0.276468601290314));
#8290=CARTESIAN_POINT('Ctrl Pts',(0.549116837182812,2.00536570374533,0.661583099652164));
#8291=CARTESIAN_POINT('Ctrl Pts',(0.167011133590032,2.07060227586673,0.842042743615258));
#8292=CARTESIAN_POINT('Ctrl Pts',(-0.21668597901319,2.12991550296718,0.840139239691205));
#8293=CARTESIAN_POINT('Ctrl Pts',(-0.56542563851628,2.18983288558837,0.670094225008614));
#8294=CARTESIAN_POINT('Ctrl Pts',(-0.808434298594091,2.25037079909405,0.362707877766159));
#8295=CARTESIAN_POINT('Ctrl Pts',(-0.895185566716189,2.31153566652781,-0.0236000562992145));
#8296=CARTESIAN_POINT('Ctrl Pts',(-0.805022512927831,2.37333259941659,-0.413465766229975));
#8297=CARTESIAN_POINT('Ctrl Pts',(-0.552281502791154,2.43576574672377,-0.728669680768865));
#8298=CARTESIAN_POINT('Ctrl Pts',(-0.143381208770228,2.50583018408946,-0.925360181836486));
#8299=CARTESIAN_POINT('Ctrl Pts',(0.369825525208484,2.58380175548622,-0.887137157875364));
#8300=CARTESIAN_POINT('Ctrl Pts',(0.814804343279841,2.66995453964888,-0.532409524853484));
#8301=CARTESIAN_POINT('Ctrl Pts',(0.970765313247155,2.74990885053001,-0.0284299122440809));
#8302=CARTESIAN_POINT('Ctrl Pts',(0.864935389584109,2.82334491449737,0.435356252438035));
#8303=CARTESIAN_POINT('Ctrl Pts',(0.596849899496631,2.88999636123757,0.773145656467097));
#8304=CARTESIAN_POINT('Ctrl Pts',(0.205293441378129,2.95718454933558,0.962873173642001));
#8305=CARTESIAN_POINT('Ctrl Pts',(-0.232943838476479,3.0248846278283,0.964194207817526));
#8306=CARTESIAN_POINT('Ctrl Pts',(-0.631388236736662,3.09306905210793,0.774108113890306));
#8307=CARTESIAN_POINT('Ctrl Pts',(-0.909907742648915,3.16170797304782,0.427832174748424));
#8308=CARTESIAN_POINT('Ctrl Pts',(-1.01149030028913,3.23076953302768,-0.00760996058240064));
#8309=CARTESIAN_POINT('Ctrl Pts',(-0.913775364912534,3.30021940688078,-0.446516565593066));
#8310=CARTESIAN_POINT('Ctrl Pts',(-0.634094793286599,3.37002153658447,-0.801516768025116));
#8311=CARTESIAN_POINT('Ctrl Pts',(-0.226357821320832,3.4401382001316,-1.00113129709783));
#8312=CARTESIAN_POINT('Ctrl Pts',(0.229385441734438,3.51053009248794,-1.00435311710641));
#8313=CARTESIAN_POINT('Ctrl Pts',(0.642894477389595,3.581156328932,-0.809062746948213));
#8314=CARTESIAN_POINT('Ctrl Pts',(0.931669474071348,3.65197488117754,-0.452972351757245));
#8315=CARTESIAN_POINT('Ctrl Pts',(1.03789787376058,3.72294319562607,-0.00578432429799382));
#8316=CARTESIAN_POINT('Ctrl Pts',(0.939501321407795,3.79401668275829,0.443524276145958));
#8317=CARTESIAN_POINT('Ctrl Pts',(0.62476031217733,3.87305514732048,0.847385644602313));
#8318=CARTESIAN_POINT('Ctrl Pts',(0.0927824485508912,3.96002981676028,1.06307663026052));
#8319=CARTESIAN_POINT('Ctrl Pts',(-0.519261103648405,4.05484139765325,0.930258619011824));
#8320=CARTESIAN_POINT('Ctrl Pts',(-0.913615764923826,4.14159563870383,0.515316188012155));
#8321=CARTESIAN_POINT('Ctrl Pts',(-1.03259539479936,4.22024766361548,0.0197349878659042));
#8322=CARTESIAN_POINT('Ctrl Pts',(-0.936985021298801,4.29082468340848,-0.426901854675045));
#8323=CARTESIAN_POINT('Ctrl Pts',(-0.657842936611053,4.36116731303318,-0.78698353983026));
#8324=CARTESIAN_POINT('Ctrl Pts',(-0.29706363491301,4.42343562231095,-0.967045529816717));
#8325=CARTESIAN_POINT('Ctrl Pts',(0.048089905369423,4.47772349208189,-0.997758532861414));
#8326=CARTESIAN_POINT('Ctrl Pts',(0.434672946626173,4.53955785964178,-0.91663997594521));
#8327=CARTESIAN_POINT('Ctrl Pts',(0.836338179989597,4.61643768531908,-0.606572728149323));
#8328=CARTESIAN_POINT('Ctrl Pts',(1.02363261661145,4.70795057452343,-0.0318742450840044));
#8329=CARTESIAN_POINT('Ctrl Pts',(0.856646027640753,4.79864210207537,0.543182406487656));
#8330=CARTESIAN_POINT('Ctrl Pts',(0.399518272233148,4.88845129456705,0.920894696277978));
#8331=CARTESIAN_POINT('Ctrl Pts',(-0.184736991833155,4.97729888029892,0.97542191054148));
#8332=CARTESIAN_POINT('Ctrl Pts',(-0.692427413956977,5.06517207449486,0.694672374006644));
#8333=CARTESIAN_POINT('Ctrl Pts',(-0.951170369249242,5.15195437290911,0.183262220477753));
#8334=CARTESIAN_POINT('Ctrl Pts',(-0.87826921068102,5.23774553596991,-0.37821229083323));
#8335=CARTESIAN_POINT('Ctrl Pts',(-0.506794241817076,5.32221810148529,-0.795337281353065));
#8336=CARTESIAN_POINT('Ctrl Pts',(0.0276185714897006,5.406047337515,-0.930628214623325));
#8337=CARTESIAN_POINT('Ctrl Pts',(0.432533063223502,5.47061960053111,-0.780638115606707));
#8338=CARTESIAN_POINT('Ctrl Pts',(0.649902755493398,5.51893798204238,-0.574289574590299));
#8339=CARTESIAN_POINT('Ctrl Pts',(0.759237064104118,5.5493319389142,-0.408764864910009));
#8340=CARTESIAN_POINT('Ctrl Pts',(0.824596080015948,5.5772473038315,-0.236380043413035));
#8341=CARTESIAN_POINT('Ctrl Pts',(0.848146928563698,5.60949307144751,-0.0738121405935497));
#8342=CARTESIAN_POINT('Ctrl Pts',(0.844064325097165,5.62115590174748,0.0669803668858104));
#8343=CARTESIAN_POINT('Ctrl Pts',(0.824845436961386,5.62418839323027,0.196889811486777));
#8344=CARTESIAN_POINT('Ctrl Pts',(0.778623685751031,5.63017376408778,0.341659870964739));
#8345=CARTESIAN_POINT('Ctrl Pts',(0.679045301159248,5.64168668150034,0.509321418625131));
#8346=CARTESIAN_POINT('Ctrl Pts',(0.504281215772623,5.65193561221424,0.6922654991445));
#8347=CARTESIAN_POINT('Ctrl Pts',(0.215920333627058,5.66826890972612,0.839327880648377));
#8348=CARTESIAN_POINT('Ctrl Pts',(-0.17059735528807,5.68539243143367,0.846555779303511));
#8349=CARTESIAN_POINT('Ctrl Pts',(-0.52074345759163,5.70377212295289,0.685690634545263));
#8350=CARTESIAN_POINT('Ctrl Pts',(-0.76497770643086,5.7214785814209,0.389076426270338));
#8351=CARTESIAN_POINT('Ctrl Pts',(-0.855376950074861,5.73939616186927,0.0169517243609489));
#8352=CARTESIAN_POINT('Ctrl Pts',(-0.774879778839863,5.75713267952773,-0.356215682043892));
#8353=CARTESIAN_POINT('Ctrl Pts',(-0.540635276851386,5.77486575773549,-0.656201303963563));
#8354=CARTESIAN_POINT('Ctrl Pts',(-0.200120542834017,5.79252128061077,-0.823432503136215));
#8355=CARTESIAN_POINT('Ctrl Pts',(0.178054805747909,5.8101288140521,-0.825978016619043));
#8356=CARTESIAN_POINT('Ctrl Pts',(0.518555465070368,5.82768087002016,-0.663820021983919));
#8357=CARTESIAN_POINT('Ctrl Pts',(0.714370484503248,5.84226048424649,-0.419381891085474));
#8358=CARTESIAN_POINT('Ctrl Pts',(0.795543670584242,5.85390333769986,-0.187643319757738));
#8359=CARTESIAN_POINT('Ctrl Pts',(0.809262236615181,5.85970651710405,-0.067017040736679));
#8360=CARTESIAN_POINT('Ctrl Pts',(0.809328501647431,5.8626211186406,-0.00524322405284286));
#8361=CARTESIAN_POINT('Ctrl Pts',(0.761047787275267,0.0865318839626108,
-0.00420496941242302));
#8362=CARTESIAN_POINT('Ctrl Pts',(0.760985430150483,0.0892745999444253,
0.0539258014575904));
#8363=CARTESIAN_POINT('Ctrl Pts',(0.748119724422766,0.0947160261358312,
0.167035838010278));
#8364=CARTESIAN_POINT('Ctrl Pts',(0.671994482225062,0.105632770703035,0.384332182947992));
#8365=CARTESIAN_POINT('Ctrl Pts',(0.489222617092547,0.119226067914075,0.612118953075658));
#8366=CARTESIAN_POINT('Ctrl Pts',(0.173126210138464,0.135516755152735,0.762481827893436));
#8367=CARTESIAN_POINT('Ctrl Pts',(-0.17591786072793,0.151764656414447,0.759870679153006));
#8368=CARTESIAN_POINT('Ctrl Pts',(-0.488518080787529,0.167976188775447,
0.60615013690747));
#8369=CARTESIAN_POINT('Ctrl Pts',(-0.702300823925886,0.184164859419497,
0.331985628674946));
#8370=CARTESIAN_POINT('Ctrl Pts',(-0.775245837906118,0.20027867376939,-0.00713875728997948));
#8371=CARTESIAN_POINT('Ctrl Pts',(-0.693331186380063,0.216456574823254,
-0.343586819420473));
#8372=CARTESIAN_POINT('Ctrl Pts',(-0.473431441508657,0.232378967624498,
-0.610158028488542));
#8373=CARTESIAN_POINT('Ctrl Pts',(-0.160033292746761,0.248749689057296,
-0.754231386377503));
#8374=CARTESIAN_POINT('Ctrl Pts',(0.184381060038689,0.264211029038414,-0.747212343204508));
#8375=CARTESIAN_POINT('Ctrl Pts',(0.439494987793935,0.278562347450618,-0.617438290361299));
#8376=CARTESIAN_POINT('Ctrl Pts',(0.594761749184093,0.287671299007321,-0.454293092965716));
#8377=CARTESIAN_POINT('Ctrl Pts',(0.680179375188791,0.297642085136332,-0.311159344468621));
#8378=CARTESIAN_POINT('Ctrl Pts',(0.72410263440118,0.303148875483543,-0.17497012052153));
#8379=CARTESIAN_POINT('Ctrl Pts',(0.739436405987218,0.305864048225509,-0.065903096066576));
#8380=CARTESIAN_POINT('Ctrl Pts',(0.742714414172589,0.31452571142108,0.0400611631273491));
#8381=CARTESIAN_POINT('Ctrl Pts',(0.723921821344288,0.341324092131815,0.176490370677569));
#8382=CARTESIAN_POINT('Ctrl Pts',(0.663642989059462,0.367388684091378,0.335525251497113));
#8383=CARTESIAN_POINT('Ctrl Pts',(0.572000817055734,0.392510940637376,0.472934409398862));
#8384=CARTESIAN_POINT('Ctrl Pts',(0.41054956588088,0.428642412363889,0.626837468469602));
#8385=CARTESIAN_POINT('Ctrl Pts',(0.15354749226292,0.471323551336263,0.742522500650089));
#8386=CARTESIAN_POINT('Ctrl Pts',(-0.184911165258365,0.52423475364142,0.734508163497739));
#8387=CARTESIAN_POINT('Ctrl Pts',(-0.435471199252404,0.56738518488992,0.606191945550898));
#8388=CARTESIAN_POINT('Ctrl Pts',(-0.588079297608022,0.602267720216433,
0.446158216855588));
#8389=CARTESIAN_POINT('Ctrl Pts',(-0.701585525374809,0.637046993340004,
0.256315862648341));
#8390=CARTESIAN_POINT('Ctrl Pts',(-0.758246999238167,0.680601831991576,
-0.0198107154225673));
#8391=CARTESIAN_POINT('Ctrl Pts',(-0.67581747589741,0.732951768293531,-0.348648501705937));
#8392=CARTESIAN_POINT('Ctrl Pts',(-0.458356924520715,0.785453130585882,
-0.609932960571064));
#8393=CARTESIAN_POINT('Ctrl Pts',(-0.148060077521017,0.8381505627929,-0.75180328824606));
#8394=CARTESIAN_POINT('Ctrl Pts',(0.194648602326754,0.891090429842906,-0.74518574293805));
#8395=CARTESIAN_POINT('Ctrl Pts',(0.502306763187505,0.944317348882362,-0.589925789789185));
#8396=CARTESIAN_POINT('Ctrl Pts',(0.713634675628132,0.997875028872795,-0.315003755248991));
#8397=CARTESIAN_POINT('Ctrl Pts',(0.785485102314095,1.051805127184,0.0266887056339002));
#8398=CARTESIAN_POINT('Ctrl Pts',(0.701568173162039,1.10614794715317,0.368370321572409));
#8399=CARTESIAN_POINT('Ctrl Pts',(0.476045494703238,1.1609417180984,0.642213034060343));
#8400=CARTESIAN_POINT('Ctrl Pts',(0.151284968811604,1.21622234017789,0.792632503395218));
#8401=CARTESIAN_POINT('Ctrl Pts',(-0.20994906929914,1.27202327147521,0.787444219944241));
#8402=CARTESIAN_POINT('Ctrl Pts',(-0.536462340262496,1.32837570512521,0.624662675732468));
#8403=CARTESIAN_POINT('Ctrl Pts',(-0.762505777513781,1.38530791222031,0.333519162029373));
#8404=CARTESIAN_POINT('Ctrl Pts',(-0.840905814264777,1.4428452883087,-0.0306479907520013));
#8405=CARTESIAN_POINT('Ctrl Pts',(-0.752819154390827,1.50101033643261,-0.396772374613101));
#8406=CARTESIAN_POINT('Ctrl Pts',(-0.512148554946034,1.55982256369068,-0.691829494739243));
#8407=CARTESIAN_POINT('Ctrl Pts',(-0.163487647715867,1.61929805770311,-0.855273682981701));
#8408=CARTESIAN_POINT('Ctrl Pts',(0.225906877040415,1.67944986134947,-0.85149921851126));
#8409=CARTESIAN_POINT('Ctrl Pts',(0.540022411129438,1.73352770394763,-0.696678959007169));
#8410=CARTESIAN_POINT('Ctrl Pts',(0.745035426037874,1.78129469019987,-0.47100411639915));
#8411=CARTESIAN_POINT('Ctrl Pts',(0.895228236006619,1.83629699527816,-0.153554506686288));
#8412=CARTESIAN_POINT('Ctrl Pts',(0.89223927295861,1.90582241797352,0.305405109016149));
#8413=CARTESIAN_POINT('Ctrl Pts',(0.601186880623915,1.98342811819678,0.726898276477956));
#8414=CARTESIAN_POINT('Ctrl Pts',(0.182706367734971,2.05486560581464,0.924537453077089));
#8415=CARTESIAN_POINT('Ctrl Pts',(-0.237609869111216,2.11983305006345,0.922431795780973));
#8416=CARTESIAN_POINT('Ctrl Pts',(-0.619591863889922,2.18545817037548,0.736139114456955));
#8417=CARTESIAN_POINT('Ctrl Pts',(-0.885570229363876,2.25172476080031,0.399599069489404));
#8418=CARTESIAN_POINT('Ctrl Pts',(-0.980372360862589,2.31861247300258,-0.0228969605362083));
#8419=CARTESIAN_POINT('Ctrl Pts',(-0.881808807432037,2.38609753937237,-0.448648878205793));
#8420=CARTESIAN_POINT('Ctrl Pts',(-0.606198581990288,2.45415533882294,-0.792189601098245));
#8421=CARTESIAN_POINT('Ctrl Pts',(-0.161322178004925,2.53037145581947,-1.00603161350487));
#8422=CARTESIAN_POINT('Ctrl Pts',(0.395299379371196,2.61494109989725,-0.964252877413945));
#8423=CARTESIAN_POINT('Ctrl Pts',(0.875781410044385,2.70801792789744,-0.580702867265662));
#8424=CARTESIAN_POINT('Ctrl Pts',(1.04313455820602,2.79401491131878,-0.0385318102786846));
#8425=CARTESIAN_POINT('Ctrl Pts',(0.929559356135266,2.87266356126334,0.458076873271283));
#8426=CARTESIAN_POINT('Ctrl Pts',(0.643431418456286,2.94376259155564,0.81825259369129));
#8427=CARTESIAN_POINT('Ctrl Pts',(0.227420031512275,3.0151340339755,1.01956294456111));
#8428=CARTESIAN_POINT('Ctrl Pts',(-0.236013305313231,3.08673230669762,1.02071321244897));
#8429=CARTESIAN_POINT('Ctrl Pts',(-0.655312712092223,3.15851088990362,0.82039134401966));
#8430=CARTESIAN_POINT('Ctrl Pts',(-0.946873850914351,3.23042227399561,0.457473966449741));
#8431=CARTESIAN_POINT('Ctrl Pts',(-1.05249407916205,3.3024186749887,0.00351263177645307));
#8432=CARTESIAN_POINT('Ctrl Pts',(-0.950881505784981,3.37445127017033,-0.451603133534446));
#8433=CARTESIAN_POINT('Ctrl Pts',(-0.662123411549799,3.44647137006206,-0.81766079968186));
#8434=CARTESIAN_POINT('Ctrl Pts',(-0.243599361895897,3.51843039638608,-1.02223134291874));
#8435=CARTESIAN_POINT('Ctrl Pts',(0.221519869149556,3.59028009019258,-1.02522354552454));
#8436=CARTESIAN_POINT('Ctrl Pts',(0.641079480627667,3.66197241810962,-0.826743985088088));
#8437=CARTESIAN_POINT('Ctrl Pts',(0.932305753772203,3.73346042815455,-0.467154572986677));
#8438=CARTESIAN_POINT('Ctrl Pts',(1.03861864013118,3.80469836360394,-0.0182689927929131));
#8439=CARTESIAN_POINT('Ctrl Pts',(0.940131774495132,3.87564133945326,0.430064269101829));
#8440=CARTESIAN_POINT('Ctrl Pts',(0.627502787803768,3.95409130409743,0.830659036467112));
#8441=CARTESIAN_POINT('Ctrl Pts',(0.102830685831636,4.03984100530226,1.04268581584403));
#8442=CARTESIAN_POINT('Ctrl Pts',(-0.49583525761956,4.13261541880481,0.912068995906106));
#8443=CARTESIAN_POINT('Ctrl Pts',(-0.878366090562576,4.21687097129819,0.508686580065169));
#8444=CARTESIAN_POINT('Ctrl Pts',(-0.992885546867205,4.29278745506574,0.0303715986090578));
#8445=CARTESIAN_POINT('Ctrl Pts',(-0.900857732990206,4.36055726365513,-0.398358938076031));
#8446=CARTESIAN_POINT('Ctrl Pts',(-0.634099084538523,4.42774028194511,-0.742056089518087));
#8447=CARTESIAN_POINT('Ctrl Pts',(-0.291218725591637,4.48691789775377,-0.912954776843569));
#8448=CARTESIAN_POINT('Ctrl Pts',(0.0353338389981778,4.53828673655579,-0.941939927553755));
#8449=CARTESIAN_POINT('Ctrl Pts',(0.399935353975762,4.59661294894598,-0.865337605334092));
#8450=CARTESIAN_POINT('Ctrl Pts',(0.776733005244855,4.66879116737576,-0.573932764898443));
#8451=CARTESIAN_POINT('Ctrl Pts',(0.951069874501058,4.75420618445989,-0.0374521233468979));
#8452=CARTESIAN_POINT('Ctrl Pts',(0.795667633690238,4.83839691545189,0.496192145698146));
#8453=CARTESIAN_POINT('Ctrl Pts',(0.37321551266873,4.92135696236781,0.844777150582056));
#8454=CARTESIAN_POINT('Ctrl Pts',(-0.164103030175536,5.00307222290658,0.89459526891222));
#8455=CARTESIAN_POINT('Ctrl Pts',(-0.629072367177604,5.0835808762759,0.637182693614477));
#8456=CARTESIAN_POINT('Ctrl Pts',(-0.865197189154805,5.16284198642629,0.170019140261218));
#8457=CARTESIAN_POINT('Ctrl Pts',(-0.798632160692577,5.24101666855333,-0.341498002751401));
#8458=CARTESIAN_POINT('Ctrl Pts',(-0.460704756527705,5.31784810950332,-0.720915681127745));
#8459=CARTESIAN_POINT('Ctrl Pts',(0.0250637377885678,5.39406441483692,-0.843757665617551));
#8460=CARTESIAN_POINT('Ctrl Pts',(0.392990376745248,5.45271234048302,-0.707685397427104));
#8461=CARTESIAN_POINT('Ctrl Pts',(0.590886086419297,5.49672449031458,-0.519704269941511));
#8462=CARTESIAN_POINT('Ctrl Pts',(0.690089356012577,5.52426320420706,-0.369685469098573));
#8463=CARTESIAN_POINT('Ctrl Pts',(0.749986856847359,5.54988405732148,-0.211693609781653));
#8464=CARTESIAN_POINT('Ctrl Pts',(0.771247480786565,5.5791110781329,-0.0641437187273063));
#8465=CARTESIAN_POINT('Ctrl Pts',(0.767559108577705,5.5895217918739,0.0617789617871054));
#8466=CARTESIAN_POINT('Ctrl Pts',(0.750267438830112,5.59229078540417,0.1793701629056));
#8467=CARTESIAN_POINT('Ctrl Pts',(0.707806638640959,5.59776618035719,0.312188989757919));
#8468=CARTESIAN_POINT('Ctrl Pts',(0.617454783946614,5.60822690750947,0.464239989617154));
#8469=CARTESIAN_POINT('Ctrl Pts',(0.458222505179838,5.61756366364294,0.631003603405752));
#8470=CARTESIAN_POINT('Ctrl Pts',(0.195608798086434,5.63243894035577,0.764899762204783));
#8471=CARTESIAN_POINT('Ctrl Pts',(-0.156734375337364,5.64804714333712,0.771570078046333));
#8472=CARTESIAN_POINT('Ctrl Pts',(-0.476157477378167,5.66481182477952,0.624830251716582));
#8473=CARTESIAN_POINT('Ctrl Pts',(-0.699166641732472,5.68097672133402,0.354063891223433));
#8474=CARTESIAN_POINT('Ctrl Pts',(-0.781809684955192,5.69734721833354,0.0140380494345926));
#8475=CARTESIAN_POINT('Ctrl Pts',(-0.708225911167346,5.71356808697831,-0.327254794077137));
#8476=CARTESIAN_POINT('Ctrl Pts',(-0.493842847323202,5.72979893847812,-0.601910253289176));
#8477=CARTESIAN_POINT('Ctrl Pts',(-0.181803249930931,5.74597891382901,-0.755179002729622));
#8478=CARTESIAN_POINT('Ctrl Pts',(0.165081534768499,5.76212746374758,-0.757603397746925));
#8479=CARTESIAN_POINT('Ctrl Pts',(0.477820093240158,5.77824890979495,-0.608663812994026));
#8480=CARTESIAN_POINT('Ctrl Pts',(0.6578420250033,5.79164639431488,-0.38407899922635));
#8481=CARTESIAN_POINT('Ctrl Pts',(0.73258150965522,5.80236905918813,-0.170643907361132));
#8482=CARTESIAN_POINT('Ctrl Pts',(0.745186517603766,5.80770263705373,-0.0597742556711138));
#8483=CARTESIAN_POINT('Ctrl Pts',(0.7452477302825,5.81039501584596,-0.00271036138976081));
#8484=CARTESIAN_POINT('Ctrl Pts',(0.73637554456597,-0.034905906819044,0.00149822141910957));
#8485=CARTESIAN_POINT('Ctrl Pts',(0.736315065289215,-0.0322457861110944,
0.0578784184156994));
#8486=CARTESIAN_POINT('Ctrl Pts',(0.723855119649765,-0.0269785274444079,
0.167359731425993));
#8487=CARTESIAN_POINT('Ctrl Pts',(0.650028605659854,-0.0163885254876421,
0.37813983377051));
#8488=CARTESIAN_POINT('Ctrl Pts',(0.472321434225028,-0.00316501922295564,
0.599771077878032));
#8489=CARTESIAN_POINT('Ctrl Pts',(0.163871505776916,0.0127358734384148,
0.746643302062296));
#8490=CARTESIAN_POINT('Ctrl Pts',(-0.178020717494399,0.0286528420536995,
0.744244506328574));
#8491=CARTESIAN_POINT('Ctrl Pts',(-0.485310363153547,0.0445873742153369,
0.593274343279024));
#8492=CARTESIAN_POINT('Ctrl Pts',(-0.696321638562055,0.0605616885113584,
0.32292679089595));
#8493=CARTESIAN_POINT('Ctrl Pts',(-0.768671245607247,0.0765142879587451,
-0.0127547002843979));
#8494=CARTESIAN_POINT('Ctrl Pts',(-0.687406440746895,0.0925926786917108,
-0.346990712173085));
#8495=CARTESIAN_POINT('Ctrl Pts',(-0.468335089496597,0.108466807087251,
-0.612908749333903));
#8496=CARTESIAN_POINT('Ctrl Pts',(-0.154680439727662,0.124863290065507,
-0.757028315693898));
#8497=CARTESIAN_POINT('Ctrl Pts',(0.190960702616625,0.140381605561349,-0.750372135885658));
#8498=CARTESIAN_POINT('Ctrl Pts',(0.448402540405941,0.154868135339886,-0.619139543588245));
#8499=CARTESIAN_POINT('Ctrl Pts',(0.604563248996462,0.164038317486862,-0.455526063286282));
#8500=CARTESIAN_POINT('Ctrl Pts',(0.692801505132577,0.174257916716736,-0.30711527132824));
#8501=CARTESIAN_POINT('Ctrl Pts',(0.734793387939577,0.17965293624963,-0.175936136859199));
#8502=CARTESIAN_POINT('Ctrl Pts',(0.751540048894326,0.18236990875335,-0.0613882223735424));
#8503=CARTESIAN_POINT('Ctrl Pts',(0.7551152768952,0.192373536659344,0.0597671766645886));
#8504=CARTESIAN_POINT('Ctrl Pts',(0.734520628825619,0.220811715526587,0.203550786591925));
#8505=CARTESIAN_POINT('Ctrl Pts',(0.675504633847438,0.246103680576316,0.35918132189048));
#8506=CARTESIAN_POINT('Ctrl Pts',(0.578868420457559,0.272865433995542,0.505257411901041));
#8507=CARTESIAN_POINT('Ctrl Pts',(0.412986321050612,0.309852623360966,0.6626116128106));
#8508=CARTESIAN_POINT('Ctrl Pts',(0.143629214933139,0.354778069813508,0.785256875260767));
#8509=CARTESIAN_POINT('Ctrl Pts',(-0.213273382019863,0.410462823966773,
0.776304802181754));
#8510=CARTESIAN_POINT('Ctrl Pts',(-0.481071653546511,0.456621559736576,
0.640150666335757));
#8511=CARTESIAN_POINT('Ctrl Pts',(-0.645049975399408,0.494083274439161,
0.468120126704292));
#8512=CARTESIAN_POINT('Ctrl Pts',(-0.76767337587426,0.531645444367446,0.263243408444397));
#8513=CARTESIAN_POINT('Ctrl Pts',(-0.829576444241297,0.579005270485107,
-0.0369315336590326));
#8514=CARTESIAN_POINT('Ctrl Pts',(-0.739536781921683,0.636409241730255,
-0.397545468780097));
#8515=CARTESIAN_POINT('Ctrl Pts',(-0.499423699394477,0.694450871439599,
-0.686584733496388));
#8516=CARTESIAN_POINT('Ctrl Pts',(-0.154065623971144,0.753129042169855,
-0.844809002082346));
#8517=CARTESIAN_POINT('Ctrl Pts',(0.230043082427793,0.812469714610742,-0.837675208300425));
#8518=CARTESIAN_POINT('Ctrl Pts',(0.57700732934804,0.872482307649582,-0.662854788878878));
#8519=CARTESIAN_POINT('Ctrl Pts',(0.816658385667676,0.933178947324927,-0.35144538547475));
#8520=CARTESIAN_POINT('Ctrl Pts',(0.898620498059416,0.994565696397896,0.0374277419560443));
#8521=CARTESIAN_POINT('Ctrl Pts',(0.802909951920287,1.05664651863009,0.427776015744673));
#8522=CARTESIAN_POINT('Ctrl Pts',(0.544644961661021,1.11942139023705,0.741567536492036));
#8523=CARTESIAN_POINT('Ctrl Pts',(0.171851593218361,1.18288712411337,0.914331873365365));
#8524=CARTESIAN_POINT('Ctrl Pts',(-0.243417621312868,1.24703708395778,0.908422505121099));
#8525=CARTESIAN_POINT('Ctrl Pts',(-0.619017067558737,1.31186124271971,0.721193184700129));
#8526=CARTESIAN_POINT('Ctrl Pts',(-0.879004743729533,1.37734624187562,0.386310675363197));
#8527=CARTESIAN_POINT('Ctrl Pts',(-0.96906803258655,1.44347559484074,-0.0322424359567551));
#8528=CARTESIAN_POINT('Ctrl Pts',(-0.86790031511075,1.51022949541887,-0.452411800402243));
#8529=CARTESIAN_POINT('Ctrl Pts',(-0.592183196027881,1.57758514542425,-0.790265094277825));
#8530=CARTESIAN_POINT('Ctrl Pts',(-0.193888028157913,1.64551645506606,-0.976825784968679));
#8531=CARTESIAN_POINT('Ctrl Pts',(0.249421550450008,1.71399556449574,-0.972363226152577));
#8532=CARTESIAN_POINT('Ctrl Pts',(0.60558237598945,1.77532311066709,-0.796625051039305));
#8533=CARTESIAN_POINT('Ctrl Pts',(0.8371883048312,1.82929951027981,-0.541571674018944));
#8534=CARTESIAN_POINT('Ctrl Pts',(1.00631683477663,1.89125996956894,-0.183892861007664));
#8535=CARTESIAN_POINT('Ctrl Pts',(1.00242998154866,1.96919011817703,0.330561809156308));
#8536=CARTESIAN_POINT('Ctrl Pts',(0.678046985374588,2.05553891375192,0.799182526288706));
#8537=CARTESIAN_POINT('Ctrl Pts',(0.215592871821504,2.13445507623113,1.0171687785436));
#8538=CARTESIAN_POINT('Ctrl Pts',(-0.245755484917588,2.20575860450121,1.01453735558465));
#8539=CARTESIAN_POINT('Ctrl Pts',(-0.662053460345902,2.27730056442067,0.811105927156774));
#8540=CARTESIAN_POINT('Ctrl Pts',(-0.949698082269248,2.34903208294355,0.446555465549961));
#8541=CARTESIAN_POINT('Ctrl Pts',(-1.05120940332528,2.42090642547716,-0.00756626728458379));
#8542=CARTESIAN_POINT('Ctrl Pts',(-0.945694482920606,2.4928757819371,-0.4615554336784));
#8543=CARTESIAN_POINT('Ctrl Pts',(-0.65373309706183,2.5648890385768,-0.824852112339042));
#8544=CARTESIAN_POINT('Ctrl Pts',(-0.186398333660609,2.64490897695139,-1.04896208339846));
#8545=CARTESIAN_POINT('Ctrl Pts',(0.392428601415204,2.7328524366949,-1.00457390440015));
#8546=CARTESIAN_POINT('Ctrl Pts',(0.885991466423781,2.82859190723886,-0.609209043800457));
#8547=CARTESIAN_POINT('Ctrl Pts',(1.05529995356455,2.91605815749467,-0.0574670440883165));
#8548=CARTESIAN_POINT('Ctrl Pts',(0.9404267219597,2.99525759198824,0.442525460783353));
#8549=CARTESIAN_POINT('Ctrl Pts',(0.654351201989198,3.06625247050285,0.801954035756638));
#8550=CARTESIAN_POINT('Ctrl Pts',(0.242213795090643,3.13691829410408,1.0008916007729));
#8551=CARTESIAN_POINT('Ctrl Pts',(-0.212826652864091,3.20721313967166,1.0015903788085));
#8552=CARTESIAN_POINT('Ctrl Pts',(-0.620911802020433,3.27709644689386,0.806151274826951));
#8553=CARTESIAN_POINT('Ctrl Pts',(-0.902125441555246,3.346530047767,0.455442957406053));
#8554=CARTESIAN_POINT('Ctrl Pts',(-1.00288290378015,3.4154781217763,0.0205687076323444));
#8555=CARTESIAN_POINT('Ctrl Pts',(-0.905954016002294,3.48390687931578,-0.411728459241468));
#8556=CARTESIAN_POINT('Ctrl Pts',(-0.633471988666003,3.55178531279618,-0.756523888501645));
#8557=CARTESIAN_POINT('Ctrl Pts',(-0.241848429631614,3.61908513776168,-0.947526609455785));
#8558=CARTESIAN_POINT('Ctrl Pts',(0.189945078096326,3.68578091114585,-0.949941774132402));
#8559=CARTESIAN_POINT('Ctrl Pts',(0.576477351023386,3.75184999351971,-0.766702857245504));
#8560=CARTESIAN_POINT('Ctrl Pts',(0.842763477392158,3.8172729927887,-0.437388143078907));
#8561=CARTESIAN_POINT('Ctrl Pts',(0.939109365943567,3.8820336930257,-0.0292161955326936));
#8562=CARTESIAN_POINT('Ctrl Pts',(0.849864816244772,3.94611895345907,0.375744052309441));
#8563=CARTESIAN_POINT('Ctrl Pts',(0.568855507252894,4.01656349980271,0.735302720458443));
#8564=CARTESIAN_POINT('Ctrl Pts',(0.100527017909476,4.09306752580417,0.923988313796093));
#8565=CARTESIAN_POINT('Ctrl Pts',(-0.429947676508057,4.17529113638153,0.807712312565125));
#8566=CARTESIAN_POINT('Ctrl Pts',(-0.766751457693363,4.24953574058285,0.451988417955662));
#8567=CARTESIAN_POINT('Ctrl Pts',(-0.867055620215192,4.31614550668835,0.0322747096910515));
#8568=CARTESIAN_POINT('Ctrl Pts',(-0.786433787248155,4.37542306155643,-0.342717095306736));
#8569=CARTESIAN_POINT('Ctrl Pts',(-0.553591509894623,4.43404220613309,-0.642541415975661));
#8570=CARTESIAN_POINT('Ctrl Pts',(-0.254949703661647,4.48557926548469,-0.791315045323506));
#8571=CARTESIAN_POINT('Ctrl Pts',(0.0291570293227571,4.53027084332476,-0.816516772993576));
#8572=CARTESIAN_POINT('Ctrl Pts',(0.34619385996304,4.58098898265564,-0.74988353629077));
#8573=CARTESIAN_POINT('Ctrl Pts',(0.673732054403288,4.64373218633335,-0.496576750812237));
#8574=CARTESIAN_POINT('Ctrl Pts',(0.82549313959929,4.71804398143699,-0.0298835092300268));
#8575=CARTESIAN_POINT('Ctrl Pts',(0.690193167473631,4.79144721668186,0.435414793532684));
#8576=CARTESIAN_POINT('Ctrl Pts',(0.320794878503593,4.86403017533548,0.740603743058106));
#8577=CARTESIAN_POINT('Ctrl Pts',(-0.151524491360473,4.9358681380332,0.784763307633389));
#8578=CARTESIAN_POINT('Ctrl Pts',(-0.563015565921111,5.00708900174122,0.557523867207184));
#8579=CARTESIAN_POINT('Ctrl Pts',(-0.773979622003058,5.0777175836591,0.141392160563352));
#8580=CARTESIAN_POINT('Ctrl Pts',(-0.714701089250428,5.14803770018125,-0.318452831272274));
#8581=CARTESIAN_POINT('Ctrl Pts',(-0.408547263645104,5.21774614874156,-0.663787058404696));
#8582=CARTESIAN_POINT('Ctrl Pts',(0.0377467936430655,5.28789319353309,-0.776707496152719));
#8583=CARTESIAN_POINT('Ctrl Pts',(0.379199506697345,5.3421227793977,-0.652201607333827));
#8584=CARTESIAN_POINT('Ctrl Pts',(0.566192011320162,5.38383905564062,-0.473845537381084));
#8585=CARTESIAN_POINT('Ctrl Pts',(0.657798720524143,5.40903749727977,-0.33633854004436));
#8586=CARTESIAN_POINT('Ctrl Pts',(0.717053599435862,5.43460550016389,-0.179948423725179));
#8587=CARTESIAN_POINT('Ctrl Pts',(0.736001368409038,5.46142838699592,-0.0436390822672414));
#8588=CARTESIAN_POINT('Ctrl Pts',(0.732699533805117,5.47025673802722,0.0641384327733226));
#8589=CARTESIAN_POINT('Ctrl Pts',(0.717267567487411,5.4729425292515,0.172968061121252));
#8590=CARTESIAN_POINT('Ctrl Pts',(0.674294164528167,5.47835838582523,0.306417150876912));
#8591=CARTESIAN_POINT('Ctrl Pts',(0.589367588858167,5.48826679742246,0.448845634849525));
#8592=CARTESIAN_POINT('Ctrl Pts',(0.435863681849203,5.49726231481398,0.610050170577536));
#8593=CARTESIAN_POINT('Ctrl Pts',(0.183474856261557,5.51156216531003,0.738484171703071));
#8594=CARTESIAN_POINT('Ctrl Pts',(-0.15694360185226,5.5266426310904,0.745339088711981));
#8595=CARTESIAN_POINT('Ctrl Pts',(-0.466506518539338,5.54288563637211,0.603119649458923));
#8596=CARTESIAN_POINT('Ctrl Pts',(-0.683508500038263,5.55860912503815,0.339956939095868));
#8597=CARTESIAN_POINT('Ctrl Pts',(-0.76427454408521,5.57458525070198,0.00814296699892715));
#8598=CARTESIAN_POINT('Ctrl Pts',(-0.692356403067418,5.59047260948722,-0.326097245851733));
#8599=CARTESIAN_POINT('Ctrl Pts',(-0.481746476318328,5.60642757350697,-0.596113095643866));
#8600=CARTESIAN_POINT('Ctrl Pts',(-0.17408149905981,5.62238535008145,-0.747388705979419));
#8601=CARTESIAN_POINT('Ctrl Pts',(0.169257356596068,5.63837052884417,-0.749914108394102));
#8602=CARTESIAN_POINT('Ctrl Pts',(0.479957957880237,5.65438561617626,-0.602089252884573));
#8603=CARTESIAN_POINT('Ctrl Pts',(0.659507649463215,5.66774084121688,-0.378313552937684));
#8604=CARTESIAN_POINT('Ctrl Pts',(0.734262801294851,5.67846120191509,-0.164945117362021));
#8605=CARTESIAN_POINT('Ctrl Pts',(0.746897136391519,5.68380075014365,-0.0539621818883113));
#8606=CARTESIAN_POINT('Ctrl Pts',(0.746958383329741,5.68649463580539,0.00313364989116945));
#8607=CARTESIAN_POINT('Ctrl Pts',(0.815814566835808,-0.130330224170313,
0.00608572964042181));
#8608=CARTESIAN_POINT('Ctrl Pts',(0.81574777595044,-0.127392493648317,0.0683497558772952));
#8609=CARTESIAN_POINT('Ctrl Pts',(0.801917574530648,-0.121541016479789,
0.189982180475291));
#8610=CARTESIAN_POINT('Ctrl Pts',(0.720076179708318,-0.109802135369318,
0.423637133286657));
#8611=CARTESIAN_POINT('Ctrl Pts',(0.52257246527071,-0.0950959479830286,
0.670216682430069));
#8612=CARTESIAN_POINT('Ctrl Pts',(0.178979683579792,-0.0773850759889481,
0.833857879295006));
#8613=CARTESIAN_POINT('Ctrl Pts',(-0.202796111060343,-0.0596110875399413,
0.831300817004344));
#8614=CARTESIAN_POINT('Ctrl Pts',(-0.546704079234265,-0.0417815048249506,
0.662418911525214));
#8615=CARTESIAN_POINT('Ctrl Pts',(-0.783372055029714,-0.0238709819185979,
0.35933385919972));
#8616=CARTESIAN_POINT('Ctrl Pts',(-0.864753184875197,-0.00594851111055415,
-0.0178353956933698));
#8617=CARTESIAN_POINT('Ctrl Pts',(-0.773334478176264,0.0121517608065129,
-0.394117637746769));
#8618=CARTESIAN_POINT('Ctrl Pts',(-0.526336675575813,0.0300528300152245,
-0.694128101109789));
#8619=CARTESIAN_POINT('Ctrl Pts',(-0.171927989293085,0.0485816853748002,
-0.856967812451655));
#8620=CARTESIAN_POINT('Ctrl Pts',(0.219241892302673,0.0661435690780971,
-0.849629386053875));
#8621=CARTESIAN_POINT('Ctrl Pts',(0.511269538813996,0.0825752908016491,
-0.700651718265711));
#8622=CARTESIAN_POINT('Ctrl Pts',(0.688212742884786,0.0929688824026967,
-0.515482668277123));
#8623=CARTESIAN_POINT('Ctrl Pts',(0.789271830384269,0.104634211773544,-0.345264898065252));
#8624=CARTESIAN_POINT('Ctrl Pts',(0.835840552685706,0.110681117563011,-0.199292500069916));
#8625=CARTESIAN_POINT('Ctrl Pts',(0.855436969693802,0.113747420452251,-0.0672545127801751));
#8626=CARTESIAN_POINT('Ctrl Pts',(0.859596453826075,0.125693134598882,0.0768115217328358));
#8627=CARTESIAN_POINT('Ctrl Pts',(0.835580628255172,0.158478985952571,0.242058833227751));
#8628=CARTESIAN_POINT('Ctrl Pts',(0.769586439779735,0.186651953774656,0.416048967226574));
#8629=CARTESIAN_POINT('Ctrl Pts',(0.658452988538062,0.21754434815504,0.584536130831614));
#8630=CARTESIAN_POINT('Ctrl Pts',(0.469519452725492,0.259607908285106,0.763402550354253));
#8631=CARTESIAN_POINT('Ctrl Pts',(0.160734960161315,0.311184105034643,0.904533612040456));
#8632=CARTESIAN_POINT('Ctrl Pts',(-0.248644367702824,0.375004866555694,
0.893945308130918));
#8633=CARTESIAN_POINT('Ctrl Pts',(-0.556602119263691,0.428104050100634,
0.737655460917103));
#8634=CARTESIAN_POINT('Ctrl Pts',(-0.745182863285185,0.471182200071971,
0.539740059091461));
#8635=CARTESIAN_POINT('Ctrl Pts',(-0.886266592347643,0.514399233249597,
0.304055938312498));
#8636=CARTESIAN_POINT('Ctrl Pts',(-0.957458750454754,0.568882943884272,
-0.0413059341030232));
#8637=CARTESIAN_POINT('Ctrl Pts',(-0.853887718406504,0.634887576404429,
-0.455926605369635));
#8638=CARTESIAN_POINT('Ctrl Pts',(-0.578091030559718,0.701536127276082,
-0.787776294385279));
#8639=CARTESIAN_POINT('Ctrl Pts',(-0.182233203349808,0.768786900212478,
-0.96900716503876));
#8640=CARTESIAN_POINT('Ctrl Pts',(0.256863321069564,0.836623147963356,-0.960702433495544));
#8641=CARTESIAN_POINT('Ctrl Pts',(0.652172274145209,0.905012686367301,-0.761322606502187));
#8642=CARTESIAN_POINT('Ctrl Pts',(0.924097590363894,0.97392627441344,-0.407635822997762));
#8643=CARTESIAN_POINT('Ctrl Pts',(1.01653217168693,1.04332987603216,0.0320590500081477));
#8644=CARTESIAN_POINT('Ctrl Pts',(0.908582814817597,1.11318792879187,0.471232769692432));
#8645=CARTESIAN_POINT('Ctrl Pts',(0.619256634240865,1.18346212175483,0.822317334790882));
#8646=CARTESIAN_POINT('Ctrl Pts',(0.204150883899283,1.25411247134146,1.01435361293424));
#8647=CARTESIAN_POINT('Ctrl Pts',(-0.255335039468057,1.32509717724887,1.00748846785391));
#8648=CARTESIAN_POINT('Ctrl Pts',(-0.668136059212685,1.39637243934443,0.801328514209242));
#8649=CARTESIAN_POINT('Ctrl Pts',(-0.95178292376863,1.46789329716201,0.435379201029196));
#8650=CARTESIAN_POINT('Ctrl Pts',(-1.04908342032033,1.53961364173694,-0.0186107156222253));
#8651=CARTESIAN_POINT('Ctrl Pts',(-0.939782829063175,1.61148644172385,-0.470873215884411));
#8652=CARTESIAN_POINT('Ctrl Pts',(-0.64485528669132,1.68346331508962,-0.831621436646793));
#8653=CARTESIAN_POINT('Ctrl Pts',(-0.222369067997902,1.75549676069967,-1.02904638344089));
#8654=CARTESIAN_POINT('Ctrl Pts',(0.243955251242134,1.82753697804345,-1.02392596074426));
#8655=CARTESIAN_POINT('Ctrl Pts',(0.615426482313246,1.89153843647028,-0.840188966697125));
#8656=CARTESIAN_POINT('Ctrl Pts',(0.855318789869591,1.94747725405015,-0.575802063324271));
#8657=CARTESIAN_POINT('Ctrl Pts',(1.02946598525039,2.01133219243649,-0.207079962486599));
#8658=CARTESIAN_POINT('Ctrl Pts',(1.02461676742319,2.09098355290074,0.318690126147191));
#8659=CARTESIAN_POINT('Ctrl Pts',(0.696030378324876,2.17824032684713,0.791679926775));
#8660=CARTESIAN_POINT('Ctrl Pts',(0.233125707682883,2.25721084766344,1.00931797385436));
#8661=CARTESIAN_POINT('Ctrl Pts',(-0.224626745482788,2.32796519868402,1.00629897457127));
#8662=CARTESIAN_POINT('Ctrl Pts',(-0.6339746836948,2.39835286352834,0.805772864644811));
#8663=CARTESIAN_POINT('Ctrl Pts',(-0.914248320879519,2.46833600847822,0.449890991772054));
#8664=CARTESIAN_POINT('Ctrl Pts',(-1.01204327526433,2.5378754581275,0.0104708032017498));
#8665=CARTESIAN_POINT('Ctrl Pts',(-0.910398591671283,2.60693484615627,-0.425022640350768));
#8666=CARTESIAN_POINT('Ctrl Pts',(-0.632223205978339,2.67548141089082,-0.770545903348306));
#8667=CARTESIAN_POINT('Ctrl Pts',(-0.19077915573745,2.7510331430239,-0.981739247361055));
#8668=CARTESIAN_POINT('Ctrl Pts',(0.350751639619575,2.83332392956361,-0.939388071703264));
#8669=CARTESIAN_POINT('Ctrl Pts',(0.807381113276876,2.92201019365174,-0.572493800660723));
#8670=CARTESIAN_POINT('Ctrl Pts',(0.962046111870681,3.00226828074056,-0.0660538679639963));
#8671=CARTESIAN_POINT('Ctrl Pts',(0.85713814001635,3.07437416292012,0.389020737528709));
#8672=CARTESIAN_POINT('Ctrl Pts',(0.598160067164623,3.13859474978663,0.71396957225712));
#8673=CARTESIAN_POINT('Ctrl Pts',(0.227513112204098,3.20213038395221,0.892582288991036));
#8674=CARTESIAN_POINT('Ctrl Pts',(-0.179271494271356,3.2649741489312,0.892967527550594));
#8675=CARTESIAN_POINT('Ctrl Pts',(-0.542077110569308,3.32712245118683,0.718969078756907));
#8676=CARTESIAN_POINT('Ctrl Pts',(-0.790803776808349,3.38857518661434,0.408461321979562));
#8677=CARTESIAN_POINT('Ctrl Pts',(-0.879425724537882,3.44933557104976,0.0252016951514755));
#8678=CARTESIAN_POINT('Ctrl Pts',(-0.794189164113485,3.50941028939361,-0.354277655648452));
#8679=CARTESIAN_POINT('Ctrl Pts',(-0.55565506297383,3.56880938467294,-0.655921922746495));
#8680=CARTESIAN_POINT('Ctrl Pts',(-0.213823010267795,3.62754617171746,-0.822536668641497));
#8681=CARTESIAN_POINT('Ctrl Pts',(0.162262209172046,3.68563719276518,-0.824574857159711));
#8682=CARTESIAN_POINT('Ctrl Pts',(0.498443927724332,3.74310228788488,-0.665165063005605));
#8683=CARTESIAN_POINT('Ctrl Pts',(0.729881649584937,3.79996423846298,-0.378933927775719));
#8684=CARTESIAN_POINT('Ctrl Pts',(0.813641419711406,3.85624871099306,-0.0241850976803255));
#8685=CARTESIAN_POINT('Ctrl Pts',(0.736071862764344,3.91198415322131,0.328038266669519));
#8686=CARTESIAN_POINT('Ctrl Pts',(0.491395700987951,3.97333733749312,0.641249037607122));
#8687=CARTESIAN_POINT('Ctrl Pts',(0.0825465259422065,4.04013869614394,0.806230684729123));
#8688=CARTESIAN_POINT('Ctrl Pts',(-0.382721908332906,4.11224152784932,0.704620519826417));
#8689=CARTESIAN_POINT('Ctrl Pts',(-0.680039342190835,4.17771585521766,0.391187900565546));
#8690=CARTESIAN_POINT('Ctrl Pts',(-0.76929256937976,4.23681129620248,0.0188477950203028));
#8691=CARTESIAN_POINT('Ctrl Pts',(-0.697572968880325,4.28971140732258,-0.315886341619577));
#8692=CARTESIAN_POINT('Ctrl Pts',(-0.488579496968913,4.34237812445738,-0.585453783834039));
#8693=CARTESIAN_POINT('Ctrl Pts',(-0.218382589504857,4.38902064898335,-0.72035790737469));
#8694=CARTESIAN_POINT('Ctrl Pts',(0.0405292667616248,4.42974503748388,-0.743431301688004));
#8695=CARTESIAN_POINT('Ctrl Pts',(0.331059864144328,4.4762200910532,-0.682509688425359));
#8696=CARTESIAN_POINT('Ctrl Pts',(0.634311856918423,4.53422578801937,-0.448867806825259));
#8697=CARTESIAN_POINT('Ctrl Pts',(0.777308025703065,4.60380885500111,-0.0121266560714404));
#8698=CARTESIAN_POINT('Ctrl Pts',(0.649801734244585,4.67347927181515,0.42983223429034));
#8699=CARTESIAN_POINT('Ctrl Pts',(0.294762018098257,4.74336277150733,0.724467046814928));
#8700=CARTESIAN_POINT('Ctrl Pts',(-0.166668777047864,4.81354665265108,0.76865483122962));
#8701=CARTESIAN_POINT('Ctrl Pts',(-0.575369590459173,4.88419837300077,0.544172082630653));
#8702=CARTESIAN_POINT('Ctrl Pts',(-0.788825555837623,4.95530546670484,0.125518342670985));
#8703=CARTESIAN_POINT('Ctrl Pts',(-0.729195472479747,5.02721825549986,-0.344625717895169));
#8704=CARTESIAN_POINT('Ctrl Pts',(-0.412514652203176,5.0994646437749,-0.703915590092393));
#8705=CARTESIAN_POINT('Ctrl Pts',(0.057341029939602,5.17342777076928,-0.823123346482292));
#8706=CARTESIAN_POINT('Ctrl Pts',(0.421084654129107,5.23099004767544,-0.692290866908447));
#8707=CARTESIAN_POINT('Ctrl Pts',(0.623676583123104,5.27629737843684,-0.498404376340492));
#8708=CARTESIAN_POINT('Ctrl Pts',(0.720981481628271,5.30284883261904,-0.353297733729362));
#8709=CARTESIAN_POINT('Ctrl Pts',(0.787637776164054,5.33179649000212,-0.177295993368771));
#8710=CARTESIAN_POINT('Ctrl Pts',(0.807127765010578,5.36013926255724,-0.0325341715478286));
#8711=CARTESIAN_POINT('Ctrl Pts',(0.803717919008967,5.36886383773889,0.0748374563281189));
#8712=CARTESIAN_POINT('Ctrl Pts',(0.787724000780127,5.37183929103461,0.19119417816538));
#8713=CARTESIAN_POINT('Ctrl Pts',(0.738463599385226,5.37794236856336,0.343374624218365));
#8714=CARTESIAN_POINT('Ctrl Pts',(0.646480275048873,5.38873716881267,0.497186329070444));
#8715=CARTESIAN_POINT('Ctrl Pts',(0.476828824598579,5.39867186989845,0.675729029825157));
#8716=CARTESIAN_POINT('Ctrl Pts',(0.198605891064882,5.41443508721909,0.817066245403871));
#8717=CARTESIAN_POINT('Ctrl Pts',(-0.178053658883927,5.43111443103978,0.82498012601868));
#8718=CARTESIAN_POINT('Ctrl Pts',(-0.521325053956367,5.44911795950504,0.667232269677396));
#8719=CARTESIAN_POINT('Ctrl Pts',(-0.762617030947825,5.46659296431868,0.374829013448801));
#8720=CARTESIAN_POINT('Ctrl Pts',(-0.852682993465006,5.48438716420124,0.0051664039567747));
#8721=CARTESIAN_POINT('Ctrl Pts',(-0.772478321394041,5.50212402713907,-0.368037589934981));
#8722=CARTESIAN_POINT('Ctrl Pts',(-0.53691097226924,5.51997297991181,-0.670213240800697));
#8723=CARTESIAN_POINT('Ctrl Pts',(-0.191971900623107,5.53786425392876,-0.839929874217262));
#8724=CARTESIAN_POINT('Ctrl Pts',(0.193776022104325,5.55582403655017,-0.842829210365558));
#8725=CARTESIAN_POINT('Ctrl Pts',(0.543544715262778,5.57384759260338,-0.676571074022088));
#8726=CARTESIAN_POINT('Ctrl Pts',(0.746106384594806,5.58891491884207,-0.42410215662072));
#8727=CARTESIAN_POINT('Ctrl Pts',(0.830496541827838,5.6010112007023,-0.183345707690691));
#8728=CARTESIAN_POINT('Ctrl Pts',(0.844806303424896,5.6070611048039,-0.057592728256197));
#8729=CARTESIAN_POINT('Ctrl Pts',(0.844875199123982,5.61009141360481,0.00663345773004059));
#8730=CARTESIAN_POINT('Ctrl Pts',(0.939906438417177,-0.1271841600964,0.00607040646680462));
#8731=CARTESIAN_POINT('Ctrl Pts',(0.939829905991479,-0.123817957632468,
0.0774157245494413));
#8732=CARTESIAN_POINT('Ctrl Pts',(0.923862944900474,-0.117061851724138,
0.2178540076698));
#8733=CARTESIAN_POINT('Ctrl Pts',(0.829693062436053,-0.103560783790796,
0.486577094486074));
#8734=CARTESIAN_POINT('Ctrl Pts',(0.602353829492948,-0.0866284912452825,
0.770507164773516));
#8735=CARTESIAN_POINT('Ctrl Pts',(0.207228405429457,-0.066265606401215,
0.958572222843141));
#8736=CARTESIAN_POINT('Ctrl Pts',(-0.231538164597868,-0.0458367855266242,
0.955647011326686));
#8737=CARTESIAN_POINT('Ctrl Pts',(-0.626436292584032,-0.0253639739002074,
0.761654157498351));
#8738=CARTESIAN_POINT('Ctrl Pts',(-0.897962831308357,-0.00481390438675121,
0.413879414597793));
#8739=CARTESIAN_POINT('Ctrl Pts',(-0.991209135863084,0.0157318195341482,
-0.0185163756664182));
#8740=CARTESIAN_POINT('Ctrl Pts',(-0.886474071362816,0.0364604191400236,
-0.449488692149847));
#8741=CARTESIAN_POINT('Ctrl Pts',(-0.603794204103174,0.0569431903993012,
-0.792698688855432));
#8742=CARTESIAN_POINT('Ctrl Pts',(-0.198747795523654,0.078114638256149,
-0.978858885997804));
#8743=CARTESIAN_POINT('Ctrl Pts',(0.2479569333992,0.098169044818479,-0.970301533460238));
#8744=CARTESIAN_POINT('Ctrl Pts',(0.580826896807821,0.1168969127321,-0.800635303947481));
#8745=CARTESIAN_POINT('Ctrl Pts',(0.782783543487387,0.128755908416602,-0.589061191580284));
#8746=CARTESIAN_POINT('Ctrl Pts',(0.897005783332951,0.141975590455534,-0.396941572724955));
#8747=CARTESIAN_POINT('Ctrl Pts',(0.951220623434889,0.148949509586055,-0.227497964180474));
#8748=CARTESIAN_POINT('Ctrl Pts',(0.972956057301772,0.15245056068407,-0.0791516212742408));
#8749=CARTESIAN_POINT('Ctrl Pts',(0.97754652886228,0.165473006281797,0.0782497587389625));
#8750=CARTESIAN_POINT('Ctrl Pts',(0.951074314734696,0.202035990104472,0.26289373696168));
#8751=CARTESIAN_POINT('Ctrl Pts',(0.875117674322805,0.234575379297086,0.463185600964872));
#8752=CARTESIAN_POINT('Ctrl Pts',(0.750919585816,0.268975213515426,0.650931093138003));
#8753=CARTESIAN_POINT('Ctrl Pts',(0.537696047856619,0.316509625068173,0.85315710508312));
#8754=CARTESIAN_POINT('Ctrl Pts',(0.192140410745468,0.374131477487151,1.01037624365697));
#8755=CARTESIAN_POINT('Ctrl Pts',(-0.264206380811682,0.445324770140323,
0.998717987200337));
#8756=CARTESIAN_POINT('Ctrl Pts',(-0.60497909247259,0.504068055142493,0.825204449287501));
#8757=CARTESIAN_POINT('Ctrl Pts',(-0.812831910323995,0.551561950105494,
0.60706127738152));
#8758=CARTESIAN_POINT('Ctrl Pts',(-0.967790000134998,0.599037654222494,
0.348058819341403));
#8759=CARTESIAN_POINT('Ctrl Pts',(-1.04533263645627,0.6585892857431,-0.0295136425529551));
#8760=CARTESIAN_POINT('Ctrl Pts',(-0.932535340945042,0.730244323598823,
-0.479582476332701));
#8761=CARTESIAN_POINT('Ctrl Pts',(-0.635006531939138,0.802063290813462,
-0.836967292035285));
#8762=CARTESIAN_POINT('Ctrl Pts',(-0.211384495481914,0.873997036925785,
-1.03048411286453));
#8763=CARTESIAN_POINT('Ctrl Pts',(0.254709981643081,0.945997256786745,-1.02125718526525));
#8764=CARTESIAN_POINT('Ctrl Pts',(0.67084303194271,1.01801469476201,-0.810910636057396));
#8765=CARTESIAN_POINT('Ctrl Pts',(0.954585138228141,1.0900005002384,-0.441157482208363));
#8766=CARTESIAN_POINT('Ctrl Pts',(1.04994123186901,1.16190629013951,0.0145248993214667));
#8767=CARTESIAN_POINT('Ctrl Pts',(0.938591683824628,1.23368378508775,0.465709565102106));
#8768=CARTESIAN_POINT('Ctrl Pts',(0.643431339510734,1.30528535077411,0.823184446043401));
#8769=CARTESIAN_POINT('Ctrl Pts',(0.223814954443136,1.37666442496449,1.01682287715933));
#8770=CARTESIAN_POINT('Ctrl Pts',(-0.236531974525708,1.44777562939584,1.00950493693116));
#8771=CARTESIAN_POINT('Ctrl Pts',(-0.646421566503835,1.51857451620532,0.804309277608774));
#8772=CARTESIAN_POINT('Ctrl Pts',(-0.925483599505392,1.58901842308451,0.443565715500478));
#8773=CARTESIAN_POINT('Ctrl Pts',(-1.02010539289345,1.65906655902036,2.42297128055727E-5));
#8774=CARTESIAN_POINT('Ctrl Pts',(-0.913819996698292,1.7286798097062,-0.437968138571777));
#8775=CARTESIAN_POINT('Ctrl Pts',(-0.630160568699183,1.79782128167042,-0.784279189982178));
#8776=CARTESIAN_POINT('Ctrl Pts',(-0.227395315121979,1.86645611005081,-0.972046706488162));
#8777=CARTESIAN_POINT('Ctrl Pts',(0.213444128321082,1.93455302367051,-0.966813468380816));
#8778=CARTESIAN_POINT('Ctrl Pts',(0.561716935446795,1.99457711577682,-0.794168385956479));
#8779=CARTESIAN_POINT('Ctrl Pts',(0.78522515015619,2.04671554814781,-0.547659082460407));
#8780=CARTESIAN_POINT('Ctrl Pts',(0.94663695478074,2.10594250251885,-0.205550399857325));
#8781=CARTESIAN_POINT('Ctrl Pts',(0.941481597089603,2.17927874983002,0.278554385535095));
#8782=CARTESIAN_POINT('Ctrl Pts',(0.641108833826435,2.25889087391522,0.709714880954011));
#8783=CARTESIAN_POINT('Ctrl Pts',(0.221833195347442,2.33039331777189,0.906449037898222));
#8784=CARTESIAN_POINT('Ctrl Pts',(-0.190123342571746,2.39406365797347,0.90345723681407));
#8785=CARTESIAN_POINT('Ctrl Pts',(-0.556303094398879,2.45704563273878,0.723775657346073));
#8786=CARTESIAN_POINT('Ctrl Pts',(-0.805584086874686,2.51933428903179,0.406858637485983));
#8787=CARTESIAN_POINT('Ctrl Pts',(-0.89199844425266,2.58092908865271,0.017575706225503));
#8788=CARTESIAN_POINT('Ctrl Pts',(-0.802166177424502,2.64183226097443,-0.366450158389341));
#8789=CARTESIAN_POINT('Ctrl Pts',(-0.557654608477566,2.70205037551361,-0.669898112087391));
#8790=CARTESIAN_POINT('Ctrl Pts',(-0.171033852000111,2.76820620838145,-0.854685840107926));
#8791=CARTESIAN_POINT('Ctrl Pts',(0.301618002943444,2.84003274926916,-0.817487415729384));
#8792=CARTESIAN_POINT('Ctrl Pts',(0.699057776995513,2.9172448186525,-0.49794966221246));
#8793=CARTESIAN_POINT('Ctrl Pts',(0.833467046929173,2.98702269611,-0.0576334810784838));
#8794=CARTESIAN_POINT('Ctrl Pts',(0.742277817555522,3.04970582955709,0.337953463887036));
#8795=CARTESIAN_POINT('Ctrl Pts',(0.517042943018354,3.10556662329371,0.620609779563879));
#8796=CARTESIAN_POINT('Ctrl Pts',(0.19426341821801,3.16090466964743,0.776222465328461));
#8797=CARTESIAN_POINT('Ctrl Pts',(-0.160746636221079,3.21575319576163,0.776648631182202));
#8798=CARTESIAN_POINT('Ctrl Pts',(-0.478318938585645,3.27014817460386,0.624475708033388));
#8799=CARTESIAN_POINT('Ctrl Pts',(-0.696896151511846,3.324127586389,0.351843616381397));
#8800=CARTESIAN_POINT('Ctrl Pts',(-0.775245270789157,3.37773119830916,0.0137962455995873));
#8801=CARTESIAN_POINT('Ctrl Pts',(-0.699871463303963,3.43100107805136,-0.322711084842332));
#8802=CARTESIAN_POINT('Ctrl Pts',(-0.487321527970625,3.48398070238957,-0.591872409021712));
#8803=CARTESIAN_POINT('Ctrl Pts',(-0.180570652930958,3.53671489691997,-0.741676361489922));
#8804=CARTESIAN_POINT('Ctrl Pts',(0.159499801668676,3.58924970548576,-0.743804151110084));
#8805=CARTESIAN_POINT('Ctrl Pts',(0.466042924677468,3.64163244121242,-0.598790110718948));
#8806=CARTESIAN_POINT('Ctrl Pts',(0.679048172164124,3.69391101203407,-0.335874179181561));
#8807=CARTESIAN_POINT('Ctrl Pts',(0.757098987300611,3.74613352942541,-0.00685566915496274));
#8808=CARTESIAN_POINT('Ctrl Pts',(0.684780334607884,3.79834928453026,0.323157073681087));
#8809=CARTESIAN_POINT('Ctrl Pts',(0.453629101282779,3.85641345347746,0.619779787434268));
#8810=CARTESIAN_POINT('Ctrl Pts',(0.0623550725553726,3.92040805691949,0.778615434185862));
#8811=CARTESIAN_POINT('Ctrl Pts',(-0.390074273721578,3.99049207085899,0.680884262897895));
#8812=CARTESIAN_POINT('Ctrl Pts',(-0.684040858644726,4.05508469998422,0.372336294124342));
#8813=CARTESIAN_POINT('Ctrl Pts',(-0.773782047272804,4.11416918249667,0.000206877778816241));
#8814=CARTESIAN_POINT('Ctrl Pts',(-0.70167834245794,4.16766962919652,-0.338346375873826));
#8815=CARTESIAN_POINT('Ctrl Pts',(-0.488341635818142,4.2215297999684,-0.614253066244098));
#8816=CARTESIAN_POINT('Ctrl Pts',(-0.209132227965426,4.26976699194909,-0.754096345125804));
#8817=CARTESIAN_POINT('Ctrl Pts',(0.0609805405658866,4.31225648238685,-0.77830614316397));
#8818=CARTESIAN_POINT('Ctrl Pts',(0.366234247622769,4.36109387197713,-0.714482850537072));
#8819=CARTESIAN_POINT('Ctrl Pts',(0.688676175467285,4.42268467081582,-0.467077355584903));
#8820=CARTESIAN_POINT('Ctrl Pts',(0.843413801971236,4.49754516558418,0.00243899912125815));
#8821=CARTESIAN_POINT('Ctrl Pts',(0.705411783279281,4.57342125554201,0.483965394365443));
#8822=CARTESIAN_POINT('Ctrl Pts',(0.314963646473482,4.65038440706278,0.809051886098812));
#8823=CARTESIAN_POINT('Ctrl Pts',(-0.198237492464167,4.72846069412574,0.858942600748725));
#8824=CARTESIAN_POINT('Ctrl Pts',(-0.657185748993143,4.80774756578419,0.607608797061368));
#8825=CARTESIAN_POINT('Ctrl Pts',(-0.899024919928932,4.88814942720442,0.134508754564314));
#8826=CARTESIAN_POINT('Ctrl Pts',(-0.831643421949731,4.96996756169197,-0.40042897985535));
#8827=CARTESIAN_POINT('Ctrl Pts',(-0.46987321377987,5.05256463965024,-0.811382428255479));
#8828=CARTESIAN_POINT('Ctrl Pts',(0.0690581953111297,5.1374089989059,-0.948414578263101));
#8829=CARTESIAN_POINT('Ctrl Pts',(0.487312195028491,5.20360536084171,-0.798018478839387));
#8830=CARTESIAN_POINT('Ctrl Pts',(0.720297973143596,5.25569818779602,-0.57510729034124));
#8831=CARTESIAN_POINT('Ctrl Pts',(0.832335357294807,5.28628902729891,-0.407959995971762));
#8832=CARTESIAN_POINT('Ctrl Pts',(0.908873130351851,5.31950870716802,-0.205878602913977));
#8833=CARTESIAN_POINT('Ctrl Pts',(0.931363540892335,5.35216146376384,-0.0392745058560254));
#8834=CARTESIAN_POINT('Ctrl Pts',(0.927434195664507,5.36234522228185,0.0857875461811561));
#8835=CARTESIAN_POINT('Ctrl Pts',(0.908875105564033,5.36576783693661,0.220317388486051));
#8836=CARTESIAN_POINT('Ctrl Pts',(0.852286384985471,5.37279307838038,0.395250245876621));
#8837=CARTESIAN_POINT('Ctrl Pts',(0.746062550306667,5.3852497453038,0.572917610790592));
#8838=CARTESIAN_POINT('Ctrl Pts',(0.550528031875155,5.39670172092908,0.77866612250797));
#8839=CARTESIAN_POINT('Ctrl Pts',(0.229815579370894,5.41487269450219,0.941605990938079));
#8840=CARTESIAN_POINT('Ctrl Pts',(-0.204110926197266,5.43408899022989,0.950683299904042));
#8841=CARTESIAN_POINT('Ctrl Pts',(-0.599371245479392,5.45482050028233,0.769034187245812));
#8842=CARTESIAN_POINT('Ctrl Pts',(-0.87702867899364,5.4749305717571,0.432514158981164));
#8843=CARTESIAN_POINT('Ctrl Pts',(-0.980583112087856,5.49539534630079,0.00737562741174088));
#8844=CARTESIAN_POINT('Ctrl Pts',(-0.888377645682189,5.51577904421374,-0.42153230387796));
#8845=CARTESIAN_POINT('Ctrl Pts',(-0.617828895808705,5.53627666571285,-0.76851148836897));
#8846=CARTESIAN_POINT('Ctrl Pts',(-0.222024165532676,5.5568042851676,-0.963242492518997));
#8847=CARTESIAN_POINT('Ctrl Pts',(0.22023538052913,5.57739671760846,-0.966476782276498));
#8848=CARTESIAN_POINT('Ctrl Pts',(0.620798780318651,5.59803503608039,-0.77611093732286));
#8849=CARTESIAN_POINT('Ctrl Pts',(0.85258883077245,5.61528501724234,-0.487001575340435));
#8850=CARTESIAN_POINT('Ctrl Pts',(0.949002234587475,5.62910083396811,-0.212024071906503));
#8851=CARTESIAN_POINT('Ctrl Pts',(0.965390060580142,5.6360317010903,-0.0679575811816029));
#8852=CARTESIAN_POINT('Ctrl Pts',(0.965468448539529,5.63947951751958,0.00511751240862206));
#8853=CARTESIAN_POINT('Ctrl Pts',(1.01541404854081,-0.0286935421156315,
0.00150443648987817));
#8854=CARTESIAN_POINT('Ctrl Pts',(1.0153316720095,-0.0250702924914887,0.0782977665694167));
#8855=CARTESIAN_POINT('Ctrl Pts',(0.998061067965302,-0.01776881642298,0.230061020652479));
#8856=CARTESIAN_POINT('Ctrl Pts',(0.896507970410834,-0.00321644170734523,
0.519681530472795));
#8857=CARTESIAN_POINT('Ctrl Pts',(0.651700399400465,0.0150138989322842,
0.825300432454518));
#8858=CARTESIAN_POINT('Ctrl Pts',(0.227375973227118,0.036878832048787,1.02708251861184));
#8859=CARTESIAN_POINT('Ctrl Pts',(-0.242679375804631,0.0587675112003217,
1.02386206441447));
#8860=CARTESIAN_POINT('Ctrl Pts',(-0.664613500907547,0.0806464126928114,
0.816420272619932));
#8861=CARTESIAN_POINT('Ctrl Pts',(-0.954028936186183,0.102560724404933,
0.445560203245322));
#8862=CARTESIAN_POINT('Ctrl Pts',(-1.05305061430877,0.124415052527098,-0.0143232362366139));
#8863=CARTESIAN_POINT('Ctrl Pts',(-0.941823920774565,0.146408467527581,
-0.471556911983546));
#8864=CARTESIAN_POINT('Ctrl Pts',(-0.642485376190151,0.168092546430336,
-0.834629545979693));
#8865=CARTESIAN_POINT('Ctrl Pts',(-0.214891649867034,0.190440095097436,
-1.03118613926827));
#8866=CARTESIAN_POINT('Ctrl Pts',(0.255634621569918,0.211565709991131,-1.02177602841285));
#8867=CARTESIAN_POINT('Ctrl Pts',(0.604967188378009,0.231223905635136,-0.843971173664312));
#8868=CARTESIAN_POINT('Ctrl Pts',(0.817375614875641,0.243692331658102,-0.620966234628241));
#8869=CARTESIAN_POINT('Ctrl Pts',(0.93521991933766,0.257410231695498,-0.423284374065397));
#8870=CARTESIAN_POINT('Ctrl Pts',(0.994404452315675,0.264894384309915,-0.239303687432268));
#8871=CARTESIAN_POINT('Ctrl Pts',(1.01596215324894,0.268591201966757,-0.0880723640353921));
#8872=CARTESIAN_POINT('Ctrl Pts',(1.0205039746406,0.281019326474854,0.0630908513062379));
#8873=CARTESIAN_POINT('Ctrl Pts',(0.994378414321425,0.317957096714928,0.250530420627939));
#8874=CARTESIAN_POINT('Ctrl Pts',(0.912951430370462,0.353072056425804,0.465323791815171));
#8875=CARTESIAN_POINT('Ctrl Pts',(0.786921615932354,0.38772781696553,0.654734433319484));
#8876=CARTESIAN_POINT('Ctrl Pts',(0.566396891602532,0.437024433912912,0.864633138859578));
#8877=CARTESIAN_POINT('Ctrl Pts',(0.214287136160365,0.495563811300856,1.02349076931142));
#8878=CARTESIAN_POINT('Ctrl Pts',(-0.248413771213054,0.567872730344711,
1.01212656684935));
#8879=CARTESIAN_POINT('Ctrl Pts',(-0.590158481993694,0.626768703811191,
0.837169097794829));
#8880=CARTESIAN_POINT('Ctrl Pts',(-0.797510277958299,0.674174341970158,
0.619616869419747));
#8881=CARTESIAN_POINT('Ctrl Pts',(-0.951354574490064,0.721326912001104,
0.36226182871036));
#8882=CARTESIAN_POINT('Ctrl Pts',(-1.02758183833276,0.780135727695703,-0.0105470253631208));
#8883=CARTESIAN_POINT('Ctrl Pts',(-0.916742267762083,0.850265458962013,
-0.450941013164969));
#8884=CARTESIAN_POINT('Ctrl Pts',(-0.627617874156891,0.919998168879143,
-0.79759899354444));
#8885=CARTESIAN_POINT('Ctrl Pts',(-0.219645029295957,0.989251615618451,
-0.983505765471186));
#8886=CARTESIAN_POINT('Ctrl Pts',(0.225381885584275,1.05801068462552,-0.974300058686517));
#8887=CARTESIAN_POINT('Ctrl Pts',(0.619361047095629,1.12623348932208,-0.774713667806041));
#8888=CARTESIAN_POINT('Ctrl Pts',(0.885716095501334,1.19389398672781,-0.426999836263685));
#8889=CARTESIAN_POINT('Ctrl Pts',(0.974291026212976,1.26096321722367,-0.00195020977515301));
#8890=CARTESIAN_POINT('Ctrl Pts',(0.870876015266758,1.32741755937141,0.415634325020865));
#8891=CARTESIAN_POINT('Ctrl Pts',(0.599338144996461,1.39323527154609,0.743980912787849));
#8892=CARTESIAN_POINT('Ctrl Pts',(0.216180250636426,1.45839836163331,0.920451353607443));
#8893=CARTESIAN_POINT('Ctrl Pts',(-0.201272117097304,1.52289181314394,0.913522853159369));
#8894=CARTESIAN_POINT('Ctrl Pts',(-0.570548639662344,1.58670389932783,0.728354841003099));
#8895=CARTESIAN_POINT('Ctrl Pts',(-0.820382402521458,1.64982630148298,0.404986062705005));
#8896=CARTESIAN_POINT('Ctrl Pts',(-0.904479685668547,1.71225408373635,0.00968826999415909));
#8897=CARTESIAN_POINT('Ctrl Pts',(-0.810038574444765,1.7739857088511,-0.378630014114413));
#8898=CARTESIAN_POINT('Ctrl Pts',(-0.559509437490529,1.8350230574724,-0.684209923886114));
#8899=CARTESIAN_POINT('Ctrl Pts',(-0.205333854139325,1.89537153055327,-0.849154186548771));
#8900=CARTESIAN_POINT('Ctrl Pts',(0.180913185811132,1.95503963034863,-0.844441083709361));
#8901=CARTESIAN_POINT('Ctrl Pts',(0.485145501820239,2.00748431759449,-0.693529326700443));
#8902=CARTESIAN_POINT('Ctrl Pts',(0.680025653214346,2.05294977689377,-0.4785681353795));
#8903=CARTESIAN_POINT('Ctrl Pts',(0.820569325450077,2.10453041033964,-0.180613181464698));
#8904=CARTESIAN_POINT('Ctrl Pts',(0.816018280899283,2.16830917571319,0.240386482303728));
#8905=CARTESIAN_POINT('Ctrl Pts',(0.554982945114321,2.23749424473742,0.615072637612301));
#8906=CARTESIAN_POINT('Ctrl Pts',(0.190474109677823,2.29966157986966,0.786172683784692));
#8907=CARTESIAN_POINT('Ctrl Pts',(-0.16810567273515,2.35508007174548,0.783641241011412));
#8908=CARTESIAN_POINT('Ctrl Pts',(-0.487480644144325,2.41000246178756,0.627042764779694));
#8909=CARTESIAN_POINT('Ctrl Pts',(-0.705547500524523,2.46446249857771,0.350025298859625));
#8910=CARTESIAN_POINT('Ctrl Pts',(-0.781519650084714,2.51849770387977,0.00853405927247853));
#8911=CARTESIAN_POINT('Ctrl Pts',(-0.702570992198226,2.57214827844602,-0.329827714267465));
#8912=CARTESIAN_POINT('Ctrl Pts',(-0.486274342611164,2.62545312866023,-0.59860543001831));
#8913=CARTESIAN_POINT('Ctrl Pts',(-0.142162838703697,2.68435626813191,-0.763377855466168));
#8914=CARTESIAN_POINT('Ctrl Pts',(0.281841368907173,2.74877887629358,-0.73060196102912));
#8915=CARTESIAN_POINT('Ctrl Pts',(0.642352611343018,2.81872244827704,-0.441705029191515));
#8916=CARTESIAN_POINT('Ctrl Pts',(0.766135230581646,2.88262056243045,-0.0386487887714388));
#8917=CARTESIAN_POINT('Ctrl Pts',(0.682146453828098,2.94061856579323,0.327550649434606));
#8918=CARTESIAN_POINT('Ctrl Pts',(0.471988991973713,2.99280172387605,0.591860756051737));
#8919=CARTESIAN_POINT('Ctrl Pts',(0.167546526079099,3.04501676534233,0.739073495501827));
#8920=CARTESIAN_POINT('Ctrl Pts',(-0.171001703799227,3.09731247177318,0.739884148714911));
#8921=CARTESIAN_POINT('Ctrl Pts',(-0.477304502784758,3.14973690901181,0.593577403675705));
#8922=CARTESIAN_POINT('Ctrl Pts',(-0.690674180169148,3.20233769539631,0.328129045034359));
#8923=CARTESIAN_POINT('Ctrl Pts',(-0.768323012250615,3.25516121598218,-0.00496084478245173));
#8924=CARTESIAN_POINT('Ctrl Pts',(-0.693617521096008,3.30825337771062,-0.340504233555695));
#8925=CARTESIAN_POINT('Ctrl Pts',(-0.479667676648141,3.36165845234506,-0.612152379685385));
#8926=CARTESIAN_POINT('Ctrl Pts',(-0.167078917313426,3.41541915108854,-0.765297478660572));
#8927=CARTESIAN_POINT('Ctrl Pts',(0.183558850259758,3.46957641471836,-0.767927865892618));
#8928=CARTESIAN_POINT('Ctrl Pts',(0.503285298567085,3.52416949866324,-0.617153128637687));
#8929=CARTESIAN_POINT('Ctrl Pts',(0.728015013291304,3.57923520646701,-0.340429122081529));
#8930=CARTESIAN_POINT('Ctrl Pts',(0.811494657084915,3.63480791389034,0.00967126530056645));
#8931=CARTESIAN_POINT('Ctrl Pts',(0.734134654405728,3.69091962908469,0.364469200185399));
#8932=CARTESIAN_POINT('Ctrl Pts',(0.483731297324057,3.75389710925618,0.686496005848039));
#8933=CARTESIAN_POINT('Ctrl Pts',(0.0551920067279564,3.82402651455037,0.861293716109767));
#8934=CARTESIAN_POINT('Ctrl Pts',(-0.446129312901893,3.90164697131953,0.753780321290741));
#8935=CARTESIAN_POINT('Ctrl Pts',(-0.775266770278101,3.97386573112298,0.409205356780351));
#8936=CARTESIAN_POINT('Ctrl Pts',(-0.876587779067353,4.04038539752733,-0.00977508211755218));
#8937=CARTESIAN_POINT('Ctrl Pts',(-0.795163896594075,4.10093301846076,-0.393025295166194));
#8938=CARTESIAN_POINT('Ctrl Pts',(-0.552701413631269,4.16217441976383,-0.706895391311044));
#8939=CARTESIAN_POINT('Ctrl Pts',(-0.234038723763906,4.21722706264337,-0.866632297588611));
#8940=CARTESIAN_POINT('Ctrl Pts',(0.0751068254044917,4.26585255357816,-0.894373061766401));
#8941=CARTESIAN_POINT('Ctrl Pts',(0.42505471576597,4.32183524942327,-0.821248980428701));
#8942=CARTESIAN_POINT('Ctrl Pts',(0.795538664900941,4.39258201646211,-0.53714913283713));
#8943=CARTESIAN_POINT('Ctrl Pts',(0.973592661579039,4.47869159574723,0.00294967027693707));
#8944=CARTESIAN_POINT('Ctrl Pts',(0.814764167968699,4.56598160688673,0.556927408855015));
#8945=CARTESIAN_POINT('Ctrl Pts',(0.365947861529639,4.65442275123741,0.93038704854384));
#8946=CARTESIAN_POINT('Ctrl Pts',(-0.222497764166292,4.74394347109101,0.98733029944098));
#8947=CARTESIAN_POINT('Ctrl Pts',(-0.746767612105839,4.83453546306066,0.69978571984963));
#8948=CARTESIAN_POINT('Ctrl Pts',(-1.02143955519273,4.9260176862291,0.161418306938975));
#8949=CARTESIAN_POINT('Ctrl Pts',(-0.944719913007531,5.01856725062234,-0.443919063426878));
#8950=CARTESIAN_POINT('Ctrl Pts',(-0.537274670503414,5.11151402622739,-0.905277409599477));
#8951=CARTESIAN_POINT('Ctrl Pts',(0.0642159068265587,5.20609904237226,-1.0582150867811));
#8952=CARTESIAN_POINT('Ctrl Pts',(0.528130756131502,5.27971987016299,-0.889732582513035));
#8953=CARTESIAN_POINT('Ctrl Pts',(0.783429970494387,5.33668529254443,-0.646138507796482));
#8954=CARTESIAN_POINT('Ctrl Pts',(0.908143095679349,5.37096072629315,-0.459096780980709));
#8955=CARTESIAN_POINT('Ctrl Pts',(0.989605658092228,5.40613046868718,-0.244086405525751));
#8956=CARTESIAN_POINT('Ctrl Pts',(1.01529199200331,5.44263887842801,-0.0586913908545394));
#8957=CARTESIAN_POINT('Ctrl Pts',(1.01082053212328,5.45474573741654,0.0888385633722979));
#8958=CARTESIAN_POINT('Ctrl Pts',(0.989621265793943,5.45843623062483,0.238512855713079));
#8959=CARTESIAN_POINT('Ctrl Pts',(0.930168823774541,5.46592421796278,0.423104870225524));
#8960=CARTESIAN_POINT('Ctrl Pts',(0.813228983696787,5.4795677442685,0.619152823787792));
#8961=CARTESIAN_POINT('Ctrl Pts',(0.601537180242377,5.49197366268454,0.841509797706045));
#8962=CARTESIAN_POINT('Ctrl Pts',(0.253625678769957,5.51168590377359,1.01850144143581));
#8963=CARTESIAN_POINT('Ctrl Pts',(-0.215557143609538,5.53247096280752,1.02795739263416));
#8964=CARTESIAN_POINT('Ctrl Pts',(-0.642009135344561,5.55484828747929,0.831989439847644));
#8965=CARTESIAN_POINT('Ctrl Pts',(-0.940774441608774,5.57649768588922,0.469624887452474));
#8966=CARTESIAN_POINT('Ctrl Pts',(-1.05185609843952,5.59848042348958,0.0130672783119852));
#8967=CARTESIAN_POINT('Ctrl Pts',(-0.95294724142773,5.6203207553287,-0.446431339614107));
#8968=CARTESIAN_POINT('Ctrl Pts',(-0.663635568817441,5.64223553779152,-0.817195637636098));
#8969=CARTESIAN_POINT('Ctrl Pts',(-0.241597801203389,5.66412201642128,-1.02472095530409));
#8970=CARTESIAN_POINT('Ctrl Pts',(0.228854601267908,5.68603053593709,-1.02797194332589));
#8971=CARTESIAN_POINT('Ctrl Pts',(0.65379320906392,5.70792720813883,-0.825928779568734));
#8972=CARTESIAN_POINT('Ctrl Pts',(0.899104794299161,5.72619390359354,-0.519721925751465));
#8973=CARTESIAN_POINT('Ctrl Pts',(1.00091159660272,5.74078191241576,-0.229396086229819));
#8974=CARTESIAN_POINT('Ctrl Pts',(1.01823042784667,5.74810326039065,-0.0772232183289336));
#8975=CARTESIAN_POINT('Ctrl Pts',(1.01831301276113,5.75173567571447,-0.000235624821140368));
#8976=CARTESIAN_POINT('Ctrl Pts',(0.984648983550121,0.0916287761618602,
-0.00420559214620277));
#8977=CARTESIAN_POINT('Ctrl Pts',(0.984569074047288,0.0951435159976226,
0.070287916264845));
#8978=CARTESIAN_POINT('Ctrl Pts',(0.96785159059107,0.102215071827367,0.217284031811231));
#8979=CARTESIAN_POINT('Ctrl Pts',(0.869509369496233,0.116307240942699,0.497768770660214));
#8980=CARTESIAN_POINT('Ctrl Pts',(0.632970632528384,0.133912282411646,0.792860122220623));
#8981=CARTESIAN_POINT('Ctrl Pts',(0.224010397149195,0.154982246000659,0.987232026634351));
#8982=CARTESIAN_POINT('Ctrl Pts',(-0.227738935737947,0.176014947093011,
0.983956925535199));
#8983=CARTESIAN_POINT('Ctrl Pts',(-0.632225622436782,0.196990217342226,
0.784980269761374));
#8984=CARTESIAN_POINT('Ctrl Pts',(-0.908833156779193,0.217937334695042,
0.430268392775773));
#8985=CARTESIAN_POINT('Ctrl Pts',(-1.00315714269518,0.238779889329383,-0.00839180413288515));
#8986=CARTESIAN_POINT('Ctrl Pts',(-0.897234292107521,0.259696501114417,
-0.443410759159778));
#8987=CARTESIAN_POINT('Ctrl Pts',(-0.613012989293456,0.28027363660682,-0.787843327150621));
#8988=CARTESIAN_POINT('Ctrl Pts',(-0.208321048403559,0.301410715181248,
-0.973943372778342));
#8989=CARTESIAN_POINT('Ctrl Pts',(0.236187823064961,0.321365472013982,-0.96472154867092));
#8990=CARTESIAN_POINT('Ctrl Pts',(0.564934420323231,0.339858954187646,-0.797635836250644));
#8991=CARTESIAN_POINT('Ctrl Pts',(0.765284272143534,0.351610475561473,-0.586892505079194));
#8992=CARTESIAN_POINT('Ctrl Pts',(0.874430977800043,0.364384335814288,-0.404270210132846));
#8993=CARTESIAN_POINT('Ctrl Pts',(0.932132473479406,0.37156393468169,-0.225771771401753));
#8994=CARTESIAN_POINT('Ctrl Pts',(0.951322910554871,0.375063708484045,-0.0873015561040709));
#8995=CARTESIAN_POINT('Ctrl Pts',(0.95537658577755,0.385668685648629,0.042720286905362));
#8996=CARTESIAN_POINT('Ctrl Pts',(0.932151401111379,0.419279012282826,0.21413345826893));
#8997=CARTESIAN_POINT('Ctrl Pts',(0.853913450916173,0.453214817731995,0.420579039328621));
#8998=CARTESIAN_POINT('Ctrl Pts',(0.738712459359737,0.48466333959355,0.592718978656939));
#8999=CARTESIAN_POINT('Ctrl Pts',(0.533467422810344,0.530659406988462,0.788734527193056));
#9000=CARTESIAN_POINT('Ctrl Pts',(0.210148474461089,0.584247998551829,0.933437435420979));
#9001=CARTESIAN_POINT('Ctrl Pts',(-0.213066084232724,0.650471539673848,
0.923488122281593));
#9002=CARTESIAN_POINT('Ctrl Pts',(-0.522860245212984,0.70381943751296,0.764083825730224));
#9003=CARTESIAN_POINT('Ctrl Pts',(-0.710230955483532,0.746670035618981,
0.567563588265933));
#9004=CARTESIAN_POINT('Ctrl Pts',(-0.848761892340287,0.789134351036642,
0.335658385105654));
#9005=CARTESIAN_POINT('Ctrl Pts',(-0.916893515971457,0.841853183525993,
0.00135356844800982));
#9006=CARTESIAN_POINT('Ctrl Pts',(-0.81780076857272,0.904401699226823,-0.391436604244268));
#9007=CARTESIAN_POINT('Ctrl Pts',(-0.561076476779489,0.966259749866032,
-0.698868666319774));
#9008=CARTESIAN_POINT('Ctrl Pts',(-0.200613927988294,1.02742594336109,-0.86292405532288));
#9009=CARTESIAN_POINT('Ctrl Pts',(0.190898801358669,1.08790487580521,-0.854643120270496));
#9010=CARTESIAN_POINT('Ctrl Pts',(0.536220910044881,1.14770382643931,-0.679543997807491));
#9011=CARTESIAN_POINT('Ctrl Pts',(0.768939370840714,1.20683412954839,-0.375539600166186));
#9012=CARTESIAN_POINT('Ctrl Pts',(0.84608550733363,1.26531015149593,-0.00487186504282669));
#9013=CARTESIAN_POINT('Ctrl Pts',(0.755997632036065,1.32314974933626,0.358619972297139));
#9014=CARTESIAN_POINT('Ctrl Pts',(0.51984856794744,1.38037392798047,0.644112483671553));
#9015=CARTESIAN_POINT('Ctrl Pts',(0.186797875670655,1.4370066824962,0.797492861272122));
#9016=CARTESIAN_POINT('Ctrl Pts',(-0.176167084506555,1.49307481265338,0.791485998881262));
#9017=CARTESIAN_POINT('Ctrl Pts',(-0.497595223102844,1.54860817405036,0.630362526553513));
#9018=CARTESIAN_POINT('Ctrl Pts',(-0.715487592961372,1.60363908336117,0.348459189956295));
#9019=CARTESIAN_POINT('Ctrl Pts',(-0.789099563909685,1.65820225483128,0.00294658455629332));
#9020=CARTESIAN_POINT('Ctrl Pts',(-0.706405422251732,1.71233471279791,-0.337633601053105));
#9021=CARTESIAN_POINT('Ctrl Pts',(-0.485930302287288,1.76607595930567,-0.606810242202756));
#9022=CARTESIAN_POINT('Ctrl Pts',(-0.17264525878764,1.81946665376375,-0.752921334364951));
#9023=CARTESIAN_POINT('Ctrl Pts',(0.170998393471184,1.87255006029022,-0.74894300281477));
#9024=CARTESIAN_POINT('Ctrl Pts',(0.443471026407504,1.91950038239868,-0.614029119564585));
#9025=CARTESIAN_POINT('Ctrl Pts',(0.619041287830423,1.96044279001245,-0.420489990106911));
#9026=CARTESIAN_POINT('Ctrl Pts',(0.746324423909596,2.00712483590238,-0.15090641186216));
#9027=CARTESIAN_POINT('Ctrl Pts',(0.742795882826775,2.06530367893983,0.233138381400874));
#9028=CARTESIAN_POINT('Ctrl Pts',(0.502513298903239,2.12915318805118,0.579348112036599));
#9029=CARTESIAN_POINT('Ctrl Pts',(0.16253718014326,2.18716317053762,0.739396339894856));
#9030=CARTESIAN_POINT('Ctrl Pts',(-0.17539831795519,2.23939524780309,0.73736054879534));
#9031=CARTESIAN_POINT('Ctrl Pts',(-0.479690868610869,2.29169807469187,0.588598159081229));
#9032=CARTESIAN_POINT('Ctrl Pts',(-0.689894606425972,2.34412032601839,0.322210826352658));
#9033=CARTESIAN_POINT('Ctrl Pts',(-0.764219381102178,2.39670968207434,-0.0100147764634279));
#9034=CARTESIAN_POINT('Ctrl Pts',(-0.686940088797011,2.44951251931434,-0.343092764626077));
#9035=CARTESIAN_POINT('Ctrl Pts',(-0.471963980624939,2.50257679039761,-0.61087531074171));
#9036=CARTESIAN_POINT('Ctrl Pts',(-0.125846100986523,2.56186866776871,-0.777155895496916));
#9037=CARTESIAN_POINT('Ctrl Pts',(0.306695745076419,2.62758939711501,-0.744675068695687));
#9038=CARTESIAN_POINT('Ctrl Pts',(0.680536925772417,2.69999236610502,-0.44645395946444));
#9039=CARTESIAN_POINT('Ctrl Pts',(0.811399634809351,2.76710302983079,-0.0234435082030726));
#9040=CARTESIAN_POINT('Ctrl Pts',(0.722567452530805,2.82876532932536,0.365948667491797));
#9041=CARTESIAN_POINT('Ctrl Pts',(0.497274836283305,2.88479222540301,0.649896079203092));
#9042=CARTESIAN_POINT('Ctrl Pts',(0.167565378605837,2.94138117554149,0.809752108634447));
#9043=CARTESIAN_POINT('Ctrl Pts',(-0.202514861231675,2.99855915881875,0.810987742795578));
#9044=CARTESIAN_POINT('Ctrl Pts',(-0.54024836777901,3.05635084400284,0.650034647856289));
#9045=CARTESIAN_POINT('Ctrl Pts',(-0.777439808371775,3.11477744451591,0.355437259411251));
#9046=CARTESIAN_POINT('Ctrl Pts',(-0.864538532626252,3.17385708103057,-0.0169620644579516));
#9047=CARTESIAN_POINT('Ctrl Pts',(-0.780730355879149,3.23360478205715,-0.394546823931951));
#9048=CARTESIAN_POINT('Ctrl Pts',(-0.538871430519538,3.29403218226595,-0.701989737522886));
#9049=CARTESIAN_POINT('Ctrl Pts',(-0.183675044177321,3.35514758348308,-0.876223096704092));
#9050=CARTESIAN_POINT('Ctrl Pts',(0.21641742511937,3.41695593657272,-0.879385005360802));
#9051=CARTESIAN_POINT('Ctrl Pts',(0.58244885584365,3.4794588064082,-0.70691401895504));
#9052=CARTESIAN_POINT('Ctrl Pts',(0.840377488385198,3.54265437797189,-0.389457958817879));
#9053=CARTESIAN_POINT('Ctrl Pts',(0.936379051461337,3.60653744708314,0.0129064008869146));
#9054=CARTESIAN_POINT('Ctrl Pts',(0.847406337365262,3.67109977077888,0.421057242306564));
#9055=CARTESIAN_POINT('Ctrl Pts',(0.559284515754883,3.74357723142762,0.791598570275586));
#9056=CARTESIAN_POINT('Ctrl Pts',(0.0664802120480439,3.82422657018271,0.992494006014603));
#9057=CARTESIAN_POINT('Ctrl Pts',(-0.508836939749483,3.91331939878274,0.868903160147672));
#9058=CARTESIAN_POINT('Ctrl Pts',(-0.885220448376754,3.99595408400187,0.474453579430707));
#9059=CARTESIAN_POINT('Ctrl Pts',(-1.00056529854099,4.07180730080897,-0.00329165097347213));
#9060=CARTESIAN_POINT('Ctrl Pts',(-0.907890405064184,4.14060796730828,-0.43868077322946));
#9061=CARTESIAN_POINT('Ctrl Pts',(-0.633413258504046,4.20990094390894,-0.793653263367458));
#9062=CARTESIAN_POINT('Ctrl Pts',(-0.274462526690471,4.27190716068393,-0.973358002930129));
#9063=CARTESIAN_POINT('Ctrl Pts',(0.0721614216821628,4.32643224508216,-1.00438010445284));
#9064=CARTESIAN_POINT('Ctrl Pts',(0.463151416323009,4.38898332141623,-0.922576230659944));
#9065=CARTESIAN_POINT('Ctrl Pts',(0.874381781681704,4.46758260884606,-0.60648434106529));
#9066=CARTESIAN_POINT('Ctrl Pts',(1.06980246797287,4.5624608610176,-0.0111547350400171));
#9067=CARTESIAN_POINT('Ctrl Pts',(0.895542839263134,4.65778864543642,0.593582242631324));
#9068=CARTESIAN_POINT('Ctrl Pts',(0.409432656352506,4.75346464397675,0.996900689499745));
#9069=CARTESIAN_POINT('Ctrl Pts',(-0.220974884955076,4.8493586118428,1.0569724532724));
#9070=CARTESIAN_POINT('Ctrl Pts',(-0.776343503280075,4.94539607569114,0.751232219154683));
#9071=CARTESIAN_POINT('Ctrl Pts',(-1.06353864055222,5.04137406111148,0.186094576072339));
#9072=CARTESIAN_POINT('Ctrl Pts',(-0.983004483323193,5.13736802025292,-0.442038732586129));
#9073=CARTESIAN_POINT('Ctrl Pts',(-0.563899268862914,5.23282576403033,-0.914456728983043));
#9074=CARTESIAN_POINT('Ctrl Pts',(0.0462535987950873,5.32862941387192,-1.06937942849709));
#9075=CARTESIAN_POINT('Ctrl Pts',(0.512328791044282,5.4028182967163,-0.898072195820719));
#9076=CARTESIAN_POINT('Ctrl Pts',(0.764973310859695,5.45905280441918,-0.657803543587761));
#9077=CARTESIAN_POINT('Ctrl Pts',(0.890710367977351,5.49386603690105,-0.468087075222217));
#9078=CARTESIAN_POINT('Ctrl Pts',(0.968409565374987,5.52718349212031,-0.263107453230972));
#9079=CARTESIAN_POINT('Ctrl Pts',(0.995071164043899,5.56417283457121,-0.076219039962342));
#9080=CARTESIAN_POINT('Ctrl Pts',(0.990445839819153,5.57721055288114,0.0815576822316796));
#9081=CARTESIAN_POINT('Ctrl Pts',(0.968532969593368,5.58078474935199,0.231884168081497));
#9082=CARTESIAN_POINT('Ctrl Pts',(0.912864182508467,5.58792083788095,0.405697502925931));
#9083=CARTESIAN_POINT('Ctrl Pts',(0.79685593045897,5.6013750719408,0.600721988903217));
#9084=CARTESIAN_POINT('Ctrl Pts',(0.590987347316022,5.61344502070309,0.816500282778712));
#9085=CARTESIAN_POINT('Ctrl Pts',(0.251816999969086,5.63265781325075,0.989312986130609));
#9086=CARTESIAN_POINT('Ctrl Pts',(-0.203712241550418,5.652836559154,0.998070068603191));
#9087=CARTESIAN_POINT('Ctrl Pts',(-0.61681159855121,5.67451656195012,0.80825617493892));
#9088=CARTESIAN_POINT('Ctrl Pts',(-0.905346760987353,5.69542976164301,0.45798872211099));
#9089=CARTESIAN_POINT('Ctrl Pts',(-1.01228962463618,5.71661306203865,0.017991770284493));
#9090=CARTESIAN_POINT('Ctrl Pts',(-0.917075602975552,5.73760403864021,-0.423685145857852));
#9091=CARTESIAN_POINT('Ctrl Pts',(-0.639635441889197,5.75860936766058,-0.77908140747453));
#9092=CARTESIAN_POINT('Ctrl Pts',(-0.235928437930338,5.77954061301565,-0.977430172367204));
#9093=CARTESIAN_POINT('Ctrl Pts',(0.212816369821538,5.80043496339875,-0.980446947576766));
#9094=CARTESIAN_POINT('Ctrl Pts',(0.617105887642918,5.82126950130601,-0.788055472477775));
#9095=CARTESIAN_POINT('Ctrl Pts',(0.849818947223183,5.83860198442984,-0.49741920984452));
#9096=CARTESIAN_POINT('Ctrl Pts',(0.946233465126923,5.85242411596325,-0.222305253914967));
#9097=CARTESIAN_POINT('Ctrl Pts',(0.962588059762422,5.85934575684304,-0.0784255384345603));
#9098=CARTESIAN_POINT('Ctrl Pts',(0.962666377720516,5.8627904943351,-0.00541570169036758));
#9099=CARTESIAN_POINT('Ctrl Pts',(0.90955220090418,0.125678856736808,-0.00589269379913899));
#9100=CARTESIAN_POINT('Ctrl Pts',(0.909478225648677,0.128932584618482,0.0630687703907631));
#9101=CARTESIAN_POINT('Ctrl Pts',(0.894048295886179,0.135454695280294,0.198633746114812));
#9102=CARTESIAN_POINT('Ctrl Pts',(0.803209936276703,0.148472212309086,0.457715426009415));
#9103=CARTESIAN_POINT('Ctrl Pts',(0.584980168342948,0.164709446618313,0.729811293679696));
#9104=CARTESIAN_POINT('Ctrl Pts',(0.208027170967614,0.184132547183783,0.90896385424324));
#9105=CARTESIAN_POINT('Ctrl Pts',(-0.207959759216391,0.203501125169494,
0.905893140126457));
#9106=CARTESIAN_POINT('Ctrl Pts',(-0.580071872739438,0.222800673169386,
0.722802863656692));
#9107=CARTESIAN_POINT('Ctrl Pts',(-0.834346439551474,0.242061866579171,
0.396677481020101));
#9108=CARTESIAN_POINT('Ctrl Pts',(-0.92094289121704,0.261209977709745,-0.00626201767291697));
#9109=CARTESIAN_POINT('Ctrl Pts',(-0.823680568403855,0.280412428111005,
-0.405548844365146));
#9110=CARTESIAN_POINT('Ctrl Pts',(-0.562944356772313,0.299290170930855,
-0.721426233726792));
#9111=CARTESIAN_POINT('Ctrl Pts',(-0.191976003784791,0.31866955507914,-0.89198669771893));
#9112=CARTESIAN_POINT('Ctrl Pts',(0.215171433213828,0.33694918115194,-0.883456498426514));
#9113=CARTESIAN_POINT('Ctrl Pts',(0.516068099710212,0.35388104972228,-0.730545197447956));
#9114=CARTESIAN_POINT('Ctrl Pts',(0.69948513866957,0.364640684639828,-0.537522963098884));
#9115=CARTESIAN_POINT('Ctrl Pts',(0.799020464603065,0.376306845093206,-0.37106440995685));
#9116=CARTESIAN_POINT('Ctrl Pts',(0.852211021510913,0.382906747014502,-0.206674942188407));
#9117=CARTESIAN_POINT('Ctrl Pts',(0.869552750695885,0.386118378167317,-0.0807135116177633));
#9118=CARTESIAN_POINT('Ctrl Pts',(0.873228226002728,0.395604438926807,0.0358634082412919));
#9119=CARTESIAN_POINT('Ctrl Pts',(0.852178260557866,0.42620902392069,0.192171108460186));
#9120=CARTESIAN_POINT('Ctrl Pts',(0.780192267650991,0.457471749380521,0.382133130394898));
#9121=CARTESIAN_POINT('Ctrl Pts',(0.675189726878795,0.486095153937536,0.538855525199464));
#9122=CARTESIAN_POINT('Ctrl Pts',(0.487448733465738,0.52819382223328,0.718280709852067));
#9123=CARTESIAN_POINT('Ctrl Pts',(0.192301074143443,0.577093945556737,0.850202458087255));
#9124=CARTESIAN_POINT('Ctrl Pts',(-0.194211405236157,0.63760673037774,0.841257470744877));
#9125=CARTESIAN_POINT('Ctrl Pts',(-0.477073537388488,0.686323304344046,
0.695647695880699));
#9126=CARTESIAN_POINT('Ctrl Pts',(-0.648205135382649,0.725464891967771,
0.516199282848472));
#9127=CARTESIAN_POINT('Ctrl Pts',(-0.774761683593055,0.764262912420243,
0.304335592440901));
#9128=CARTESIAN_POINT('Ctrl Pts',(-0.83712527622246,0.812496673215361,-0.00140070915450113));
#9129=CARTESIAN_POINT('Ctrl Pts',(-0.746440875151343,0.869769816513919,
-0.361038867683182));
#9130=CARTESIAN_POINT('Ctrl Pts',(-0.510939112655819,0.926556842886396,
-0.643231430899843));
#9131=CARTESIAN_POINT('Ctrl Pts',(-0.179428142008608,0.982828907729359,
-0.79421329029021));
#9132=CARTESIAN_POINT('Ctrl Pts',(0.18174936978697,1.03863921522632,-0.786712467357663));
#9133=CARTESIAN_POINT('Ctrl Pts',(0.501469893757735,1.09400777439781,-0.624757152462634));
#9134=CARTESIAN_POINT('Ctrl Pts',(0.717864370714667,1.14897277405206,-0.342352558018187));
#9135=CARTESIAN_POINT('Ctrl Pts',(0.790049385509793,1.20356691455005,0.00357612389287991));
#9136=CARTESIAN_POINT('Ctrl Pts',(0.705754196611436,1.25782823693133,0.344532532610256));
#9137=CARTESIAN_POINT('Ctrl Pts',(0.483277370716406,1.31179498215349,0.613838500779083));
#9138=CARTESIAN_POINT('Ctrl Pts',(0.167585716227014,1.3655073441895,0.759481897321007));
#9139=CARTESIAN_POINT('Ctrl Pts',(-0.178658312614736,1.41900638076518,0.754000347388005));
#9140=CARTESIAN_POINT('Ctrl Pts',(-0.487358805469693,1.4723346864654,0.599549639426908));
#9141=CARTESIAN_POINT('Ctrl Pts',(-0.698165752470841,1.52553548174234,0.32725969494298));
#9142=CARTESIAN_POINT('Ctrl Pts',(-0.770084936124923,1.57865238683387,-0.00895031380089644));
#9143=CARTESIAN_POINT('Ctrl Pts',(-0.689303462132877,1.63172997477994,-0.342877489010814));
#9144=CARTESIAN_POINT('Ctrl Pts',(-0.471811562324975,1.68481246545016,-0.60887894620495));
#9145=CARTESIAN_POINT('Ctrl Pts',(-0.160236777931869,1.73794563714968,-0.75451752224437));
#9146=CARTESIAN_POINT('Ctrl Pts',(0.184257032273775,1.79117120239166,-0.750831658503854));
#9147=CARTESIAN_POINT('Ctrl Pts',(0.45962358205835,1.83861061933306,-0.614790911954126));
#9148=CARTESIAN_POINT('Ctrl Pts',(0.638154679941761,1.88022882117527,-0.418143586816256));
#9149=CARTESIAN_POINT('Ctrl Pts',(0.768250650239937,1.92791038289434,-0.142887497408747));
#9150=CARTESIAN_POINT('Ctrl Pts',(0.765210575236715,1.98778313244085,0.252300460533073));
#9151=CARTESIAN_POINT('Ctrl Pts',(0.516123981662164,2.05410503330788,0.6122539442656));
#9152=CARTESIAN_POINT('Ctrl Pts',(0.160263722031045,2.11485118755329,0.780150477387041));
#9153=CARTESIAN_POINT('Ctrl Pts',(-0.195888391503639,2.16990388596071,0.778274632766191));
#9154=CARTESIAN_POINT('Ctrl Pts',(-0.518660047512728,2.22536566924697,0.620779215863372));
#9155=CARTESIAN_POINT('Ctrl Pts',(-0.743027269231705,2.28127313124113,0.336845813371297));
#9156=CARTESIAN_POINT('Ctrl Pts',(-0.822939493772593,2.33765555827195,-0.0192857525782725));
#9157=CARTESIAN_POINT('Ctrl Pts',(-0.739895966613412,2.39454181187788,-0.378174258410101));
#9158=CARTESIAN_POINT('Ctrl Pts',(-0.507432703799843,2.45195821290454,-0.668052190846269));
#9159=CARTESIAN_POINT('Ctrl Pts',(-0.131531364679454,2.51636641537369,-0.848855077071543));
#9160=CARTESIAN_POINT('Ctrl Pts',(0.340198775675162,2.58803340462628,-0.813744118818101));
#9161=CARTESIAN_POINT('Ctrl Pts',(0.749550293417911,2.66727724174046,-0.487526234835778));
#9162=CARTESIAN_POINT('Ctrl Pts',(0.893316574148684,2.74091681990833,-0.023366466522462));
#9163=CARTESIAN_POINT('Ctrl Pts',(0.795757990210055,2.80866966254995,0.404576874166815));
#9164=CARTESIAN_POINT('Ctrl Pts',(0.548004150809532,2.87027962092074,0.716888421623811));
#9165=CARTESIAN_POINT('Ctrl Pts',(0.185289053539309,2.93252341178201,0.892760490208275));
#9166=CARTESIAN_POINT('Ctrl Pts',(-0.22175178875163,2.99540054743711,0.894109450833571));
#9167=CARTESIAN_POINT('Ctrl Pts',(-0.592939587196475,3.0589070566873,0.717178592312595));
#9168=CARTESIAN_POINT('Ctrl Pts',(-0.853291005408645,3.12303606754463,0.393731991340956));
#9169=CARTESIAN_POINT('Ctrl Pts',(-0.948684337638334,3.18777770111288,-0.0144566266599512));
#9170=CARTESIAN_POINT('Ctrl Pts',(-0.856917921474516,3.25311897476409,-0.427457214656335));
#9171=CARTESIAN_POINT('Ctrl Pts',(-0.592906791304635,3.31904398316708,-0.762872291775904));
#9172=CARTESIAN_POINT('Ctrl Pts',(-0.206327696795635,3.38553401578509,-0.952349876980599));
#9173=CARTESIAN_POINT('Ctrl Pts',(0.227690644097483,3.45256754119835,-0.955627088535012));
#9174=CARTESIAN_POINT('Ctrl Pts',(0.623316753010274,3.52012024062849,-0.769024389527845));
#9175=CARTESIAN_POINT('Ctrl Pts',(0.900967743613051,3.58816512289236,-0.427008079610695));
#9176=CARTESIAN_POINT('Ctrl Pts',(1.00375079789027,3.65667314648915,0.00463978121626096));
#9177=CARTESIAN_POINT('Ctrl Pts',(0.908532101935272,3.72561178223024,0.440525826284625));
#9178=CARTESIAN_POINT('Ctrl Pts',(0.601976701053612,3.8026511284078,0.834343685753614));
#9179=CARTESIAN_POINT('Ctrl Pts',(0.0806362141225256,3.88792074321953,1.04632070591145));
#9180=CARTESIAN_POINT('Ctrl Pts',(-0.523620625967669,3.9815022105468,0.915840845262919));
#9181=CARTESIAN_POINT('Ctrl Pts',(-0.915935792656353,4.06771715054109,0.503867434474184));
#9182=CARTESIAN_POINT('Ctrl Pts',(-1.03518812510371,4.14634770587156,0.00846388977103227));
#9183=CARTESIAN_POINT('Ctrl Pts',(-0.939354725954324,4.21726768242631,-0.44039985190263));
#9184=CARTESIAN_POINT('Ctrl Pts',(-0.657622764287281,4.2883154938952,-0.804254512732454));
#9185=CARTESIAN_POINT('Ctrl Pts',(-0.29146462647341,4.35152846153295,-0.987256117242355));
#9186=CARTESIAN_POINT('Ctrl Pts',(0.0604069213856414,4.40687215270274,-1.01864808961705));
#9187=CARTESIAN_POINT('Ctrl Pts',(0.455817860274253,4.47011933657517,-0.935785288792637));
#9188=CARTESIAN_POINT('Ctrl Pts',(0.868997154316896,4.54914650202704,-0.617456627835253));
#9189=CARTESIAN_POINT('Ctrl Pts',(1.06333617461654,4.64382389525895,-0.0230756819531807));
#9190=CARTESIAN_POINT('Ctrl Pts',(0.890037371970145,4.73823988777768,0.575750516999619));
#9191=CARTESIAN_POINT('Ctrl Pts',(0.411621565129445,4.83230120305772,0.971758552342444));
#9192=CARTESIAN_POINT('Ctrl Pts',(-0.203757910870774,4.92589103507915,1.02970525192993));
#9193=CARTESIAN_POINT('Ctrl Pts',(-0.741665205819518,5.01895623726245,0.732797837240576));
#9194=CARTESIAN_POINT('Ctrl Pts',(-1.01747315988325,5.11132924690258,0.188632511506228));
#9195=CARTESIAN_POINT('Ctrl Pts',(-0.9398967031339,5.20307972080444,-0.411824505334644));
#9196=CARTESIAN_POINT('Ctrl Pts',(-0.541277959388034,5.29378223257878,-0.860029726746955));
#9197=CARTESIAN_POINT('Ctrl Pts',(0.0347131003179486,5.38416147101441,-1.00603962268195));
#9198=CARTESIAN_POINT('Ctrl Pts',(0.472449504710221,5.45393481550324,-0.844256072565711));
#9199=CARTESIAN_POINT('Ctrl Pts',(0.708109788427302,5.50633708994253,-0.620438326433588));
#9200=CARTESIAN_POINT('Ctrl Pts',(0.826310839284909,5.53916278990257,-0.441645104060546));
#9201=CARTESIAN_POINT('Ctrl Pts',(0.897616227875116,5.56964940189299,-0.253563543686594));
#9202=CARTESIAN_POINT('Ctrl Pts',(0.92297240476864,5.60448955322945,-0.0778455347175106));
#9203=CARTESIAN_POINT('Ctrl Pts',(0.918576908769613,5.61703094943253,0.073595424072634));
#9204=CARTESIAN_POINT('Ctrl Pts',(0.897813272525461,5.62033291313822,0.214442376647703));
#9205=CARTESIAN_POINT('Ctrl Pts',(0.84717914281391,5.62687408453863,0.372908518609524));
#9206=CARTESIAN_POINT('Ctrl Pts',(0.73902806886783,5.63938763900218,0.554930118177138));
#9207=CARTESIAN_POINT('Ctrl Pts',(0.54868329335707,5.65055047950713,0.754249110630997));
#9208=CARTESIAN_POINT('Ctrl Pts',(0.234740786310109,5.66833417008755,0.914319853294209));
#9209=CARTESIAN_POINT('Ctrl Pts',(-0.186280544388743,5.68698815338276,0.922248294213509));
#9210=CARTESIAN_POINT('Ctrl Pts',(-0.567738849793441,5.70701244501641,0.746989429520979));
#9211=CARTESIAN_POINT('Ctrl Pts',(-0.833876650451468,5.72630747686717,0.423805888181072));
#9212=CARTESIAN_POINT('Ctrl Pts',(-0.932393657693937,5.74583524156656,0.018270062398184));
#9213=CARTESIAN_POINT('Ctrl Pts',(-0.844669348182326,5.76516713174664,-0.388445981353963));
#9214=CARTESIAN_POINT('Ctrl Pts',(-0.589331567089245,5.78449854502205,-0.71541788303751));
#9215=CARTESIAN_POINT('Ctrl Pts',(-0.218194045974345,5.80374206815275,-0.897714376194275));
#9216=CARTESIAN_POINT('Ctrl Pts',(0.194035074001386,5.82293729736513,-0.900444896267203));
#9217=CARTESIAN_POINT('Ctrl Pts',(0.565131377847116,5.84206506652244,-0.723768454824322));
#9218=CARTESIAN_POINT('Ctrl Pts',(0.778569851413565,5.85796115725643,-0.457245638130952));
#9219=CARTESIAN_POINT('Ctrl Pts',(0.86699247800335,5.87063993939285,-0.20490166143947));
#9220=CARTESIAN_POINT('Ctrl Pts',(0.881970292931539,5.87697404420344,-0.0732444812903123));
#9221=CARTESIAN_POINT('Ctrl Pts',(0.882042267836621,5.88013978881747,-0.00614778728168446));
#9222=CARTESIAN_POINT('Ctrl Pts',(0.872161950711206,0.124828769264236,-0.00589269379913899));
#9223=CARTESIAN_POINT('Ctrl Pts',(0.872090904698941,0.127953657301625,0.0603380612992187));
#9224=CARTESIAN_POINT('Ctrl Pts',(0.857308714561314,0.134203213047992,0.190241275757611));
#9225=CARTESIAN_POINT('Ctrl Pts',(0.770187083636269,0.146690001256174,0.438769378299054));
#9226=CARTESIAN_POINT('Ctrl Pts',(0.560950745207346,0.162256028321672,0.699616259986153));
#9227=CARTESIAN_POINT('Ctrl Pts',(0.199511576340965,0.180880209711553,0.871422024437173));
#9228=CARTESIAN_POINT('Ctrl Pts',(-0.199312333389545,0.199448331926636,
0.868457819907934));
#9229=CARTESIAN_POINT('Ctrl Pts',(-0.556088930421348,0.217951986567579,
0.692928582783942));
#9230=CARTESIAN_POINT('Ctrl Pts',(-0.799862508003898,0.236416030436661,
0.380262416576452));
#9231=CARTESIAN_POINT('Ctrl Pts',(-0.882895646021795,0.254773193569333,
-0.0060546706614528));
#9232=CARTESIAN_POINT('Ctrl Pts',(-0.789649057445972,0.273182184223599,
-0.388883291654368));
#9233=CARTESIAN_POINT('Ctrl Pts',(-0.539659944242912,0.291280837799174,
-0.691764713311758));
#9234=CARTESIAN_POINT('Ctrl Pts',(-0.183956800223335,0.309860445327341,
-0.855316888413074));
#9235=CARTESIAN_POINT('Ctrl Pts',(0.206499015809491,0.327389549600143,-0.847162298078497));
#9236=CARTESIAN_POINT('Ctrl Pts',(0.49509577120488,0.34362645645855,-0.700495805282282));
#9237=CARTESIAN_POINT('Ctrl Pts',(0.670997034604971,0.353943958171212,-0.515417881277946));
#9238=CARTESIAN_POINT('Ctrl Pts',(0.766581438347442,0.365141873832304,-0.355537227212008));
#9239=CARTESIAN_POINT('Ctrl Pts',(0.8174676017473,0.371459915026287,-0.198233634126398));
#9240=CARTESIAN_POINT('Ctrl Pts',(0.834170515466371,0.374539492519685,-0.0771620442826736));
#9241=CARTESIAN_POINT('Ctrl Pts',(0.837719002104484,0.383704512647053,0.0354460071939376));
#9242=CARTESIAN_POINT('Ctrl Pts',(0.817405541799073,0.413175723298386,0.185924750839524));
#9243=CARTESIAN_POINT('Ctrl Pts',(0.748423543506377,0.44312071842525,0.367957985006333));
#9244=CARTESIAN_POINT('Ctrl Pts',(0.647340094288683,0.470691270109384,0.518903872562794));
#9245=CARTESIAN_POINT('Ctrl Pts',(0.466898254116811,0.511144063135416,0.691309623343175));
#9246=CARTESIAN_POINT('Ctrl Pts',(0.182800989155019,0.558222951408999,0.818397523700333));
#9247=CARTESIAN_POINT('Ctrl Pts',(-0.189545178060892,0.616501258086875,
0.809773850041606));
#9248=CARTESIAN_POINT('Ctrl Pts',(-0.462507583347405,0.663503908067788,
0.669357773844709));
#9249=CARTESIAN_POINT('Ctrl Pts',(-0.627863189228003,0.701318402481341,
0.495969553901588));
#9250=CARTESIAN_POINT('Ctrl Pts',(-0.750267427503473,0.738837453517587,
0.291088758101646));
#9251=CARTESIAN_POINT('Ctrl Pts',(-0.810712868559922,0.785528896923523,
-0.00492588128797676));
#9252=CARTESIAN_POINT('Ctrl Pts',(-0.722807305049749,0.841109138477463,
-0.35397737605765));
#9253=CARTESIAN_POINT('Ctrl Pts',(-0.493845277109899,0.896322143289524,
-0.6284699970223));
#9254=CARTESIAN_POINT('Ctrl Pts',(-0.170668331595556,0.951180240767939,
-0.77578162036287));
#9255=CARTESIAN_POINT('Ctrl Pts',(0.182411368712431,1.00572789901627,-0.768554583075931));
#9256=CARTESIAN_POINT('Ctrl Pts',(0.495894675031221,1.0599979812032,-0.609891173973463));
#9257=CARTESIAN_POINT('Ctrl Pts',(0.708755333326572,1.11403086100534,-0.332295680974433));
#9258=CARTESIAN_POINT('Ctrl Pts',(0.780070637830783,1.16786510347237,0.00885468431853584));
#9259=CARTESIAN_POINT('Ctrl Pts',(0.696791510479646,1.22154183082612,0.346232027663686));
#9260=CARTESIAN_POINT('Ctrl Pts',(0.476047266626745,1.27510240963086,0.61364355273423));
#9261=CARTESIAN_POINT('Ctrl Pts',(0.161678386661078,1.32858888114584,0.758820094473604));
#9262=CARTESIAN_POINT('Ctrl Pts',(-0.184345221885054,1.38204344182885,0.753472314023915));
#9263=CARTESIAN_POINT('Ctrl Pts',(-0.493955884546455,1.43550888318168,0.598711183433611));
#9264=CARTESIAN_POINT('Ctrl Pts',(-0.706164418456796,1.48902767046263,0.324820470310737));
#9265=CARTESIAN_POINT('Ctrl Pts',(-0.778894190579621,1.54264192169839,-0.0145743797186695));
#9266=CARTESIAN_POINT('Ctrl Pts',(-0.697192877485004,1.59639341722752,-0.352835018065878));
#9267=CARTESIAN_POINT('Ctrl Pts',(-0.476282548914222,1.65032345266182,-0.623209180930827));
#9268=CARTESIAN_POINT('Ctrl Pts',(-0.158743612035258,1.70447207761938,-0.771770092812482));
#9269=CARTESIAN_POINT('Ctrl Pts',(0.193450677004803,1.75887837965647,-0.768113401787862));
#9270=CARTESIAN_POINT('Ctrl Pts',(0.47579440943534,1.80750241451549,-0.628734440560694));
#9271=CARTESIAN_POINT('Ctrl Pts',(0.659272267850805,1.85026369378763,-0.426676852570877));
#9272=CARTESIAN_POINT('Ctrl Pts',(0.793229432459306,1.89934423589563,-0.143355198493509));
#9273=CARTESIAN_POINT('Ctrl Pts',(0.790263784307131,1.96111512092083,0.264407243055348));
#9274=CARTESIAN_POINT('Ctrl Pts',(0.532639208585251,2.02974904747753,0.637020032041957));
#9275=CARTESIAN_POINT('Ctrl Pts',(0.163609475192015,2.09273970975414,0.811198964310618));
#9276=CARTESIAN_POINT('Ctrl Pts',(-0.206325324489528,2.14991769756873,0.809290051602918));
#9277=CARTESIAN_POINT('Ctrl Pts',(-0.54210311156644,2.20760646525503,0.645493293137588));
#9278=CARTESIAN_POINT('Ctrl Pts',(-0.775793177879044,2.26582771180786,0.349801965195082));
#9279=CARTESIAN_POINT('Ctrl Pts',(-0.859118193146955,2.32460053758821,-0.0214433086745682));
#9280=CARTESIAN_POINT('Ctrl Pts',(-0.772497333242961,2.38394137391289,-0.395836964477112));
#9281=CARTESIAN_POINT('Ctrl Pts',(-0.529877815574135,2.44386394296014,-0.698375208084907));
#9282=CARTESIAN_POINT('Ctrl Pts',(-0.137454124419672,2.51110274201743,-0.887126219786336));
#9283=CARTESIAN_POINT('Ctrl Pts',(0.355020405406913,2.58592160387692,-0.85044216028401));
#9284=CARTESIAN_POINT('Ctrl Pts',(0.782180417385646,2.66862024366749,-0.50996194705241));
#9285=CARTESIAN_POINT('Ctrl Pts',(0.932029131507338,2.74541647960869,-0.0258957186176781));
#9286=CARTESIAN_POINT('Ctrl Pts',(0.830321215974015,2.81601192011723,0.419957402046343));
#9287=CARTESIAN_POINT('Ctrl Pts',(0.572400166827825,2.88014282443316,0.744989944459363));
#9288=CARTESIAN_POINT('Ctrl Pts',(0.195275509838113,2.94485897026784,0.927771382562365));
#9289=CARTESIAN_POINT('Ctrl Pts',(-0.227340767365424,3.01014754818103,0.929095017890615));
#9290=CARTESIAN_POINT('Ctrl Pts',(-0.612127646814787,3.07599293903656,0.745588291188903));
#9291=CARTESIAN_POINT('Ctrl Pts',(-0.881535208369304,3.14237676662695,0.410744646425331));
#9292=CARTESIAN_POINT('Ctrl Pts',(-0.980005185206354,3.20927820175596,-0.0110388926131081));
#9293=CARTESIAN_POINT('Ctrl Pts',(-0.885263395772081,3.27667359822412,-0.436952466191731));
#9294=CARTESIAN_POINT('Ctrl Pts',(-0.613436538369041,3.34453700325931,-0.782121048029494));
#9295=CARTESIAN_POINT('Ctrl Pts',(-0.216315847404239,3.41284022102408,-0.976638893510757));
#9296=CARTESIAN_POINT('Ctrl Pts',(0.228515688692952,3.48155290325642,-0.979879367890244));
#9297=CARTESIAN_POINT('Ctrl Pts',(0.633032334246116,3.55064249055004,-0.788946617304531));
#9298=CARTESIAN_POINT('Ctrl Pts',(0.91620307923501,3.62007471455624,-0.439929095068272));
#9299=CARTESIAN_POINT('Ctrl Pts',(1.02068551154318,3.6898138200776,-0.00055988972616793));
#9300=CARTESIAN_POINT('Ctrl Pts',(0.923874643413053,3.75982214337787,0.441983752855437));
#9301=CARTESIAN_POINT('Ctrl Pts',(0.613247660943624,3.83786518922612,0.840785019888275));
#9302=CARTESIAN_POINT('Ctrl Pts',(0.0866578234258063,3.9239844102579,1.05456997463629));
#9303=CARTESIAN_POINT('Ctrl Pts',(-0.521392660403112,4.01817435387289,0.92294994186792));
#9304=CARTESIAN_POINT('Ctrl Pts',(-0.914636612404499,4.10464567111125,0.509573712510557));
#9305=CARTESIAN_POINT('Ctrl Pts',(-1.03374180999006,4.18328650371776,0.0141535738014065));
#9306=CARTESIAN_POINT('Ctrl Pts',(-0.938026942329867,4.25404428614242,-0.433573776623787));
#9307=CARTESIAN_POINT('Ctrl Pts',(-0.657630260146868,4.32474041714926,-0.795496981882739));
#9308=CARTESIAN_POINT('Ctrl Pts',(-0.294187702113077,4.38748944604847,-0.977023505420508));
#9309=CARTESIAN_POINT('Ctrl Pts',(0.0542596632323615,4.44230054898675,-1.00807090756588));
#9310=CARTESIAN_POINT('Ctrl Pts',(0.445198581282316,4.50483969839108,-0.926094625208896));
#9311=CARTESIAN_POINT('Ctrl Pts',(0.852563310440807,4.58279123657346,-0.611941112564204));
#9312=CARTESIAN_POINT('Ctrl Pts',(1.04336115553597,4.67588518836249,-0.0274765552718303));
#9313=CARTESIAN_POINT('Ctrl Pts',(0.873243552350396,4.76843871793217,0.559396655291762));
#9314=CARTESIAN_POINT('Ctrl Pts',(0.405532574611691,4.86037265153526,0.946224142384314));
#9315=CARTESIAN_POINT('Ctrl Pts',(-0.194232561825003,4.95159408982323,1.00246182575268));
#9316=CARTESIAN_POINT('Ctrl Pts',(-0.716978005254575,5.04205915598986,0.713684974901636));
#9317=CARTESIAN_POINT('Ctrl Pts',(-0.984237521133288,5.13163619116299,0.185945073380498));
#9318=CARTESIAN_POINT('Ctrl Pts',(-0.909022704364039,5.22040809154829,-0.394980663551699));
#9319=CARTESIAN_POINT('Ctrl Pts',(-0.524008362921299,5.30799616173538,-0.827628543573509));
#9320=CARTESIAN_POINT('Ctrl Pts',(0.0311612934979211,5.39510126764713,-0.968284503878036));
#9321=CARTESIAN_POINT('Ctrl Pts',(0.452486451456519,5.46227744588555,-0.812413771015693));
#9322=CARTESIAN_POINT('Ctrl Pts',(0.678996914481602,5.51263767773254,-0.597335976683866));
#9323=CARTESIAN_POINT('Ctrl Pts',(0.792756702852497,5.54424482065645,-0.425194580715441));
#9324=CARTESIAN_POINT('Ctrl Pts',(0.861097079444627,5.57344984716716,-0.244943323368279));
#9325=CARTESIAN_POINT('Ctrl Pts',(0.885548394683697,5.6069898998326,-0.0758116878038518));
#9326=CARTESIAN_POINT('Ctrl Pts',(0.881311178103886,5.61908885250671,0.0702661570768112));
#9327=CARTESIAN_POINT('Ctrl Pts',(0.861324400417122,5.62225654974902,0.205633030471336));
#9328=CARTESIAN_POINT('Ctrl Pts',(0.812891366893097,5.62852110126019,0.357273663598819));
#9329=CARTESIAN_POINT('Ctrl Pts',(0.709033945858278,5.64053429758327,0.532105911493553));
#9330=CARTESIAN_POINT('Ctrl Pts',(0.526480038594941,5.65124067536637,0.723242801555853));
#9331=CARTESIAN_POINT('Ctrl Pts',(0.225331281496905,5.66829963228703,0.876812377650357));
#9332=CARTESIAN_POINT('Ctrl Pts',(-0.178438754359568,5.6861889761217,0.884400172818289));
#9333=CARTESIAN_POINT('Ctrl Pts',(-0.544244744848784,5.70539124964099,0.716342713969011));
#9334=CARTESIAN_POINT('Ctrl Pts',(-0.799436178683323,5.72389218103035,0.406445379440496));
#9335=CARTESIAN_POINT('Ctrl Pts',(-0.893901515434013,5.74261482334007,0.0176118727011753));
#9336=CARTESIAN_POINT('Ctrl Pts',(-0.809793026073925,5.76114914213192,-0.372336066624544));
#9337=CARTESIAN_POINT('Ctrl Pts',(-0.565009292976944,5.77968086993593,-0.685823620580416));
#9338=CARTESIAN_POINT('Ctrl Pts',(-0.209171565907703,5.79813086800354,-0.860593511818846));
#9339=CARTESIAN_POINT('Ctrl Pts',(0.186034384156284,5.8165319894943,-0.863241242665013));
#9340=CARTESIAN_POINT('Ctrl Pts',(0.541844299347737,5.83487223159308,-0.693819904186464));
#9341=CARTESIAN_POINT('Ctrl Pts',(0.746471713940332,5.85010991085684,-0.43833815015316));
#9342=CARTESIAN_POINT('Ctrl Pts',(0.831270497111571,5.86227119228351,-0.19628398706425));
#9343=CARTESIAN_POINT('Ctrl Pts',(0.845616258369985,5.86833999900766,-0.0701367303899257));
#9344=CARTESIAN_POINT('Ctrl Pts',(0.845685384742026,5.87138045372904,-0.00569550566726366));
#9345=CARTESIAN_POINT('',(0.872161950711206,0.124828769264236,-0.00589269379913899));
#9346=CARTESIAN_POINT('Origin',(0.875,0.,0.));
#9347=CARTESIAN_POINT('',(0.845685384742025,5.87138045372904,-0.00569550566726366));
#9348=CARTESIAN_POINT('Ctrl Pts',(0.872161950711206,0.124828769264236,-0.00589269379913899));
#9349=CARTESIAN_POINT('Ctrl Pts',(0.872090904698941,0.127953657301625,0.0603380612992187));
#9350=CARTESIAN_POINT('Ctrl Pts',(0.857308714561314,0.134203213047992,0.190241275757611));
#9351=CARTESIAN_POINT('Ctrl Pts',(0.770187083636269,0.146690001256174,0.438769378299054));
#9352=CARTESIAN_POINT('Ctrl Pts',(0.560950745207346,0.162256028321672,0.699616259986153));
#9353=CARTESIAN_POINT('Ctrl Pts',(0.199511576340965,0.180880209711553,0.871422024437173));
#9354=CARTESIAN_POINT('Ctrl Pts',(-0.199312333389545,0.199448331926636,
0.868457819907934));
#9355=CARTESIAN_POINT('Ctrl Pts',(-0.556088930421348,0.217951986567579,
0.692928582783942));
#9356=CARTESIAN_POINT('Ctrl Pts',(-0.799862508003898,0.236416030436661,
0.380262416576452));
#9357=CARTESIAN_POINT('Ctrl Pts',(-0.882895646021795,0.254773193569333,
-0.0060546706614528));
#9358=CARTESIAN_POINT('Ctrl Pts',(-0.789649057445972,0.273182184223599,
-0.388883291654368));
#9359=CARTESIAN_POINT('Ctrl Pts',(-0.539659944242912,0.291280837799174,
-0.691764713311758));
#9360=CARTESIAN_POINT('Ctrl Pts',(-0.183956800223335,0.309860445327341,
-0.855316888413074));
#9361=CARTESIAN_POINT('Ctrl Pts',(0.206499015809491,0.327389549600143,-0.847162298078497));
#9362=CARTESIAN_POINT('Ctrl Pts',(0.49509577120488,0.34362645645855,-0.700495805282282));
#9363=CARTESIAN_POINT('Ctrl Pts',(0.670997034604971,0.353943958171212,-0.515417881277946));
#9364=CARTESIAN_POINT('Ctrl Pts',(0.766581438347442,0.365141873832304,-0.355537227212008));
#9365=CARTESIAN_POINT('Ctrl Pts',(0.8174676017473,0.371459915026287,-0.198233634126398));
#9366=CARTESIAN_POINT('Ctrl Pts',(0.834170515466371,0.374539492519685,-0.0771620442826736));
#9367=CARTESIAN_POINT('Ctrl Pts',(0.837719002104484,0.383704512647053,0.0354460071939376));
#9368=CARTESIAN_POINT('Ctrl Pts',(0.817405541799073,0.413175723298386,0.185924750839524));
#9369=CARTESIAN_POINT('Ctrl Pts',(0.748423543506377,0.44312071842525,0.367957985006333));
#9370=CARTESIAN_POINT('Ctrl Pts',(0.647340094288683,0.470691270109384,0.518903872562794));
#9371=CARTESIAN_POINT('Ctrl Pts',(0.466898254116811,0.511144063135416,0.691309623343175));
#9372=CARTESIAN_POINT('Ctrl Pts',(0.182800989155019,0.558222951408999,0.818397523700333));
#9373=CARTESIAN_POINT('Ctrl Pts',(-0.189545178060892,0.616501258086875,
0.809773850041606));
#9374=CARTESIAN_POINT('Ctrl Pts',(-0.462507583347405,0.663503908067788,
0.669357773844709));
#9375=CARTESIAN_POINT('Ctrl Pts',(-0.627863189228003,0.701318402481341,
0.495969553901588));
#9376=CARTESIAN_POINT('Ctrl Pts',(-0.750267427503473,0.738837453517587,
0.291088758101646));
#9377=CARTESIAN_POINT('Ctrl Pts',(-0.810712868559922,0.785528896923523,
-0.00492588128797676));
#9378=CARTESIAN_POINT('Ctrl Pts',(-0.722807305049749,0.841109138477463,
-0.35397737605765));
#9379=CARTESIAN_POINT('Ctrl Pts',(-0.493845277109899,0.896322143289524,
-0.6284699970223));
#9380=CARTESIAN_POINT('Ctrl Pts',(-0.170668331595556,0.951180240767939,
-0.77578162036287));
#9381=CARTESIAN_POINT('Ctrl Pts',(0.182411368712431,1.00572789901627,-0.768554583075931));
#9382=CARTESIAN_POINT('Ctrl Pts',(0.495894675031221,1.0599979812032,-0.609891173973463));
#9383=CARTESIAN_POINT('Ctrl Pts',(0.708755333326572,1.11403086100534,-0.332295680974433));
#9384=CARTESIAN_POINT('Ctrl Pts',(0.780070637830783,1.16786510347237,0.00885468431853584));
#9385=CARTESIAN_POINT('Ctrl Pts',(0.696791510479646,1.22154183082612,0.346232027663686));
#9386=CARTESIAN_POINT('Ctrl Pts',(0.476047266626745,1.27510240963086,0.61364355273423));
#9387=CARTESIAN_POINT('Ctrl Pts',(0.161678386661078,1.32858888114584,0.758820094473604));
#9388=CARTESIAN_POINT('Ctrl Pts',(-0.184345221885054,1.38204344182885,0.753472314023915));
#9389=CARTESIAN_POINT('Ctrl Pts',(-0.493955884546455,1.43550888318168,0.598711183433611));
#9390=CARTESIAN_POINT('Ctrl Pts',(-0.706164418456796,1.48902767046263,0.324820470310737));
#9391=CARTESIAN_POINT('Ctrl Pts',(-0.778894190579621,1.54264192169839,-0.0145743797186695));
#9392=CARTESIAN_POINT('Ctrl Pts',(-0.697192877485004,1.59639341722752,-0.352835018065878));
#9393=CARTESIAN_POINT('Ctrl Pts',(-0.476282548914222,1.65032345266182,-0.623209180930827));
#9394=CARTESIAN_POINT('Ctrl Pts',(-0.158743612035258,1.70447207761938,-0.771770092812482));
#9395=CARTESIAN_POINT('Ctrl Pts',(0.193450677004803,1.75887837965647,-0.768113401787862));
#9396=CARTESIAN_POINT('Ctrl Pts',(0.47579440943534,1.80750241451549,-0.628734440560694));
#9397=CARTESIAN_POINT('Ctrl Pts',(0.659272267850805,1.85026369378763,-0.426676852570877));
#9398=CARTESIAN_POINT('Ctrl Pts',(0.793229432459306,1.89934423589563,-0.143355198493509));
#9399=CARTESIAN_POINT('Ctrl Pts',(0.790263784307131,1.96111512092083,0.264407243055348));
#9400=CARTESIAN_POINT('Ctrl Pts',(0.532639208585251,2.02974904747753,0.637020032041957));
#9401=CARTESIAN_POINT('Ctrl Pts',(0.163609475192015,2.09273970975414,0.811198964310618));
#9402=CARTESIAN_POINT('Ctrl Pts',(-0.206325324489528,2.14991769756873,0.809290051602918));
#9403=CARTESIAN_POINT('Ctrl Pts',(-0.54210311156644,2.20760646525503,0.645493293137588));
#9404=CARTESIAN_POINT('Ctrl Pts',(-0.775793177879044,2.26582771180786,0.349801965195082));
#9405=CARTESIAN_POINT('Ctrl Pts',(-0.859118193146955,2.32460053758821,-0.0214433086745682));
#9406=CARTESIAN_POINT('Ctrl Pts',(-0.772497333242961,2.38394137391289,-0.395836964477112));
#9407=CARTESIAN_POINT('Ctrl Pts',(-0.529877815574135,2.44386394296014,-0.698375208084907));
#9408=CARTESIAN_POINT('Ctrl Pts',(-0.137454124419672,2.51110274201743,-0.887126219786336));
#9409=CARTESIAN_POINT('Ctrl Pts',(0.355020405406913,2.58592160387692,-0.85044216028401));
#9410=CARTESIAN_POINT('Ctrl Pts',(0.782180417385646,2.66862024366749,-0.50996194705241));
#9411=CARTESIAN_POINT('Ctrl Pts',(0.932029131507338,2.74541647960869,-0.0258957186176781));
#9412=CARTESIAN_POINT('Ctrl Pts',(0.830321215974015,2.81601192011723,0.419957402046343));
#9413=CARTESIAN_POINT('Ctrl Pts',(0.572400166827825,2.88014282443316,0.744989944459363));
#9414=CARTESIAN_POINT('Ctrl Pts',(0.195275509838113,2.94485897026784,0.927771382562365));
#9415=CARTESIAN_POINT('Ctrl Pts',(-0.227340767365424,3.01014754818103,0.929095017890615));
#9416=CARTESIAN_POINT('Ctrl Pts',(-0.612127646814787,3.07599293903656,0.745588291188903));
#9417=CARTESIAN_POINT('Ctrl Pts',(-0.881535208369304,3.14237676662695,0.410744646425331));
#9418=CARTESIAN_POINT('Ctrl Pts',(-0.980005185206354,3.20927820175596,-0.0110388926131081));
#9419=CARTESIAN_POINT('Ctrl Pts',(-0.885263395772081,3.27667359822412,-0.436952466191731));
#9420=CARTESIAN_POINT('Ctrl Pts',(-0.613436538369041,3.34453700325931,-0.782121048029494));
#9421=CARTESIAN_POINT('Ctrl Pts',(-0.216315847404239,3.41284022102408,-0.976638893510757));
#9422=CARTESIAN_POINT('Ctrl Pts',(0.228515688692952,3.48155290325642,-0.979879367890244));
#9423=CARTESIAN_POINT('Ctrl Pts',(0.633032334246116,3.55064249055004,-0.788946617304531));
#9424=CARTESIAN_POINT('Ctrl Pts',(0.91620307923501,3.62007471455624,-0.439929095068272));
#9425=CARTESIAN_POINT('Ctrl Pts',(1.02068551154318,3.6898138200776,-0.00055988972616793));
#9426=CARTESIAN_POINT('Ctrl Pts',(0.923874643413053,3.75982214337787,0.441983752855437));
#9427=CARTESIAN_POINT('Ctrl Pts',(0.613247660943624,3.83786518922612,0.840785019888275));
#9428=CARTESIAN_POINT('Ctrl Pts',(0.0866578234258063,3.9239844102579,1.05456997463629));
#9429=CARTESIAN_POINT('Ctrl Pts',(-0.521392660403112,4.01817435387289,0.92294994186792));
#9430=CARTESIAN_POINT('Ctrl Pts',(-0.914636612404499,4.10464567111125,0.509573712510557));
#9431=CARTESIAN_POINT('Ctrl Pts',(-1.03374180999006,4.18328650371776,0.0141535738014065));
#9432=CARTESIAN_POINT('Ctrl Pts',(-0.938026942329867,4.25404428614242,-0.433573776623787));
#9433=CARTESIAN_POINT('Ctrl Pts',(-0.657630260146868,4.32474041714926,-0.795496981882739));
#9434=CARTESIAN_POINT('Ctrl Pts',(-0.294187702113077,4.38748944604847,-0.977023505420508));
#9435=CARTESIAN_POINT('Ctrl Pts',(0.0542596632323615,4.44230054898675,-1.00807090756588));
#9436=CARTESIAN_POINT('Ctrl Pts',(0.445198581282316,4.50483969839108,-0.926094625208896));
#9437=CARTESIAN_POINT('Ctrl Pts',(0.852563310440807,4.58279123657346,-0.611941112564204));
#9438=CARTESIAN_POINT('Ctrl Pts',(1.04336115553597,4.67588518836249,-0.0274765552718303));
#9439=CARTESIAN_POINT('Ctrl Pts',(0.873243552350396,4.76843871793217,0.559396655291762));
#9440=CARTESIAN_POINT('Ctrl Pts',(0.405532574611691,4.86037265153526,0.946224142384314));
#9441=CARTESIAN_POINT('Ctrl Pts',(-0.194232561825003,4.95159408982323,1.00246182575268));
#9442=CARTESIAN_POINT('Ctrl Pts',(-0.716978005254575,5.04205915598986,0.713684974901636));
#9443=CARTESIAN_POINT('Ctrl Pts',(-0.984237521133288,5.13163619116299,0.185945073380498));
#9444=CARTESIAN_POINT('Ctrl Pts',(-0.909022704364039,5.22040809154829,-0.394980663551699));
#9445=CARTESIAN_POINT('Ctrl Pts',(-0.524008362921299,5.30799616173538,-0.827628543573509));
#9446=CARTESIAN_POINT('Ctrl Pts',(0.0311612934979211,5.39510126764713,-0.968284503878036));
#9447=CARTESIAN_POINT('Ctrl Pts',(0.452486451456519,5.46227744588555,-0.812413771015693));
#9448=CARTESIAN_POINT('Ctrl Pts',(0.678996914481602,5.51263767773254,-0.597335976683866));
#9449=CARTESIAN_POINT('Ctrl Pts',(0.792756702852497,5.54424482065645,-0.425194580715441));
#9450=CARTESIAN_POINT('Ctrl Pts',(0.861097079444627,5.57344984716716,-0.244943323368279));
#9451=CARTESIAN_POINT('Ctrl Pts',(0.885548394683697,5.6069898998326,-0.0758116878038518));
#9452=CARTESIAN_POINT('Ctrl Pts',(0.881311178103886,5.61908885250671,0.0702661570768112));
#9453=CARTESIAN_POINT('Ctrl Pts',(0.861324400417122,5.62225654974902,0.205633030471336));
#9454=CARTESIAN_POINT('Ctrl Pts',(0.812891366893097,5.62852110126019,0.357273663598819));
#9455=CARTESIAN_POINT('Ctrl Pts',(0.709033945858278,5.64053429758327,0.532105911493553));
#9456=CARTESIAN_POINT('Ctrl Pts',(0.526480038594941,5.65124067536637,0.723242801555853));
#9457=CARTESIAN_POINT('Ctrl Pts',(0.225331281496905,5.66829963228703,0.876812377650357));
#9458=CARTESIAN_POINT('Ctrl Pts',(-0.178438754359568,5.6861889761217,0.884400172818289));
#9459=CARTESIAN_POINT('Ctrl Pts',(-0.544244744848784,5.70539124964099,0.716342713969011));
#9460=CARTESIAN_POINT('Ctrl Pts',(-0.799436178683323,5.72389218103035,0.406445379440496));
#9461=CARTESIAN_POINT('Ctrl Pts',(-0.893901515434013,5.74261482334007,0.0176118727011753));
#9462=CARTESIAN_POINT('Ctrl Pts',(-0.809793026073925,5.76114914213192,-0.372336066624544));
#9463=CARTESIAN_POINT('Ctrl Pts',(-0.565009292976944,5.77968086993593,-0.685823620580416));
#9464=CARTESIAN_POINT('Ctrl Pts',(-0.209171565907703,5.79813086800354,-0.860593511818846));
#9465=CARTESIAN_POINT('Ctrl Pts',(0.186034384156284,5.8165319894943,-0.863241242665013));
#9466=CARTESIAN_POINT('Ctrl Pts',(0.541844299347737,5.83487223159308,-0.693819904186464));
#9467=CARTESIAN_POINT('Ctrl Pts',(0.746471713940332,5.85010991085684,-0.43833815015316));
#9468=CARTESIAN_POINT('Ctrl Pts',(0.831270497111571,5.86227119228351,-0.19628398706425));
#9469=CARTESIAN_POINT('Ctrl Pts',(0.845616258369985,5.86833999900766,-0.0701367303899257));
#9470=CARTESIAN_POINT('Ctrl Pts',(0.845685384742026,5.87138045372904,-0.00569550566726366));
#9471=CARTESIAN_POINT('Origin',(0.875,5.74999999999999,1.53717316653257E-13));
#9472=CARTESIAN_POINT('Origin',(0.875,5.74999999999999,1.53717316653257E-13));
#9473=CARTESIAN_POINT('Origin',(0.875,0.,0.));
#10249=UNCERTAINTY_MEASURE_WITH_UNIT(LENGTH_MEASURE(0.001),#10293,
'DISTANCE_ACCURACY_VALUE',
'Maximum model space distance between geometric entities at asserted c
onnectivities');
#10264=UNCERTAINTY_MEASURE_WITH_UNIT(LENGTH_MEASURE(0.001),#10293,
'DISTANCE_ACCURACY_VALUE',
'Maximum model space distance between geometric entities at asserted c
onnectivities');
#10277=(
GEOMETRIC_REPRESENTATION_CONTEXT(3)
GLOBAL_UNCERTAINTY_ASSIGNED_CONTEXT((#10249))
GLOBAL_UNIT_ASSIGNED_CONTEXT((#10293,#10295,#10296))
REPRESENTATION_CONTEXT('','3D')
);
#10292=(
GEOMETRIC_REPRESENTATION_CONTEXT(3)
GLOBAL_UNCERTAINTY_ASSIGNED_CONTEXT((#10264))
GLOBAL_UNIT_ASSIGNED_CONTEXT((#10293,#10295,#10296))
REPRESENTATION_CONTEXT('','3D')
);
#10293=(
LENGTH_UNIT()
NAMED_UNIT(*)
SI_UNIT(.CENTI.,.METRE.)
);
#10295=(
NAMED_UNIT(*)
PLANE_ANGLE_UNIT()
SI_UNIT($,.RADIAN.)
);
#10296=(
NAMED_UNIT(*)
SI_UNIT($,.STERADIAN.)
SOLID_ANGLE_UNIT()
);
#10309=SHAPE_DEFINITION_REPRESENTATION(#10336,#10425);
#10336=PRODUCT_DEFINITION_SHAPE('',$,#10453);
#10425=SHAPE_REPRESENTATION('',(#5530),#10277);
#10440=PRODUCT_DEFINITION_CONTEXT('part definition',#10523,'design');
#10453=PRODUCT_DEFINITION('Compression Spring - 2.5 mm Wire, 20 mm Outside Diameter, 60 mm Long',
'Compression Spring - 2.5 mm Wire, 20 mm Outside Diameter, 60 mm Long',
#10480,#10440);
#10480=PRODUCT_DEFINITION_FORMATION('',$,#10537);
#10523=APPLICATION_CONTEXT(
'Core Data for Automotive Mechanical Design Process');
#10524=PRODUCT_CONTEXT('part definition',#10523,'mechanical');
#10537=PRODUCT('Compression Spring - 2.5 mm Wire, 20 mm Outside Diameter, 60 mm Long',
'Compression Spring - 2.5 mm Wire, 20 mm Outside Diameter, 60 mm Long',
'Compression Spring - 2.5 mm Wire, 20 mm Outside Diameter, 60 mm Long',
(#10524));
#10622=COLOUR_RGB('Grey',0.48,0.52,0.57);
#10623=FILL_AREA_STYLE_COLOUR('',#10622);
#10624=FILL_AREA_STYLE('',(#10623));
#10625=SURFACE_STYLE_FILL_AREA(#10624);
#10626=SURFACE_SIDE_STYLE('',(#10625));
#10627=SURFACE_STYLE_USAGE(.BOTH.,#10626);
#10628=PRESENTATION_STYLE_ASSIGNMENT((#10627));
ENDSEC;
END-ISO-10303-21;
